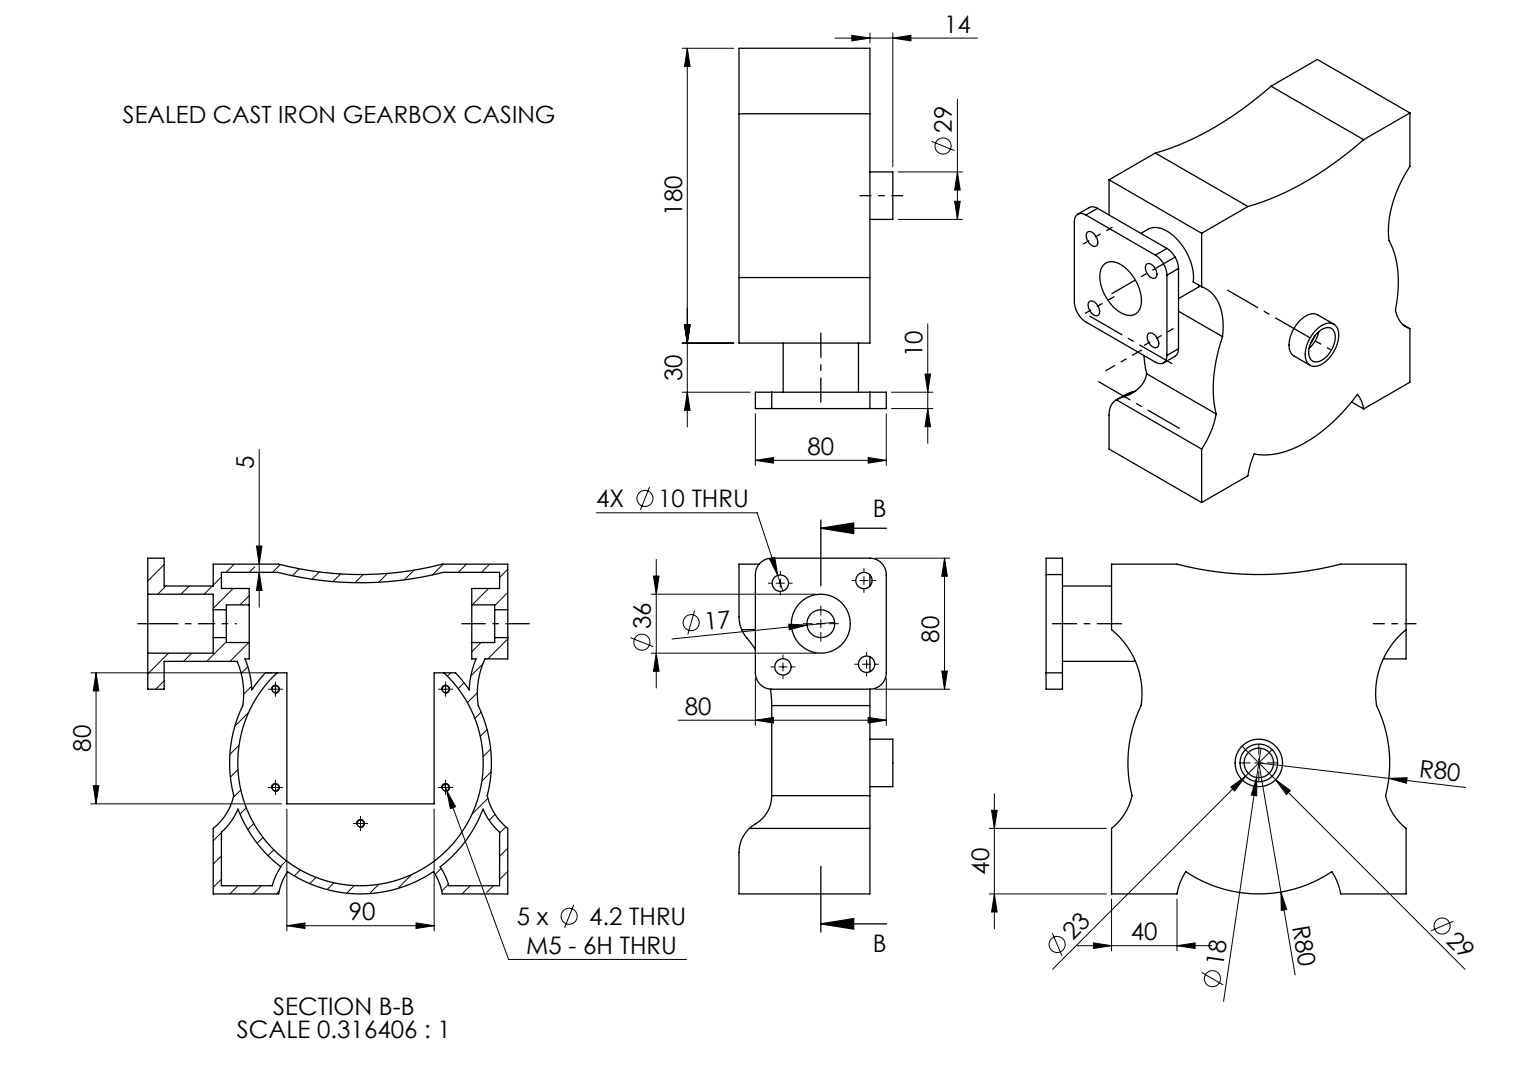
ISO-10303-21;
HEADER;
FILE_DESCRIPTION (('STEP AP214'),
    '1' );
FILE_NAME ('Sealed Cast Iron Gearbox Casing.step',
    '2026-10-03T12:29:21',
    ( '' ),
    ( '' ),
    'SwSTEP 2.0',
    'SolidWorks 2026',
    '' );
FILE_SCHEMA (( 'AUTOMOTIVE_DESIGN' ));
ENDSEC;

DATA;
#3=ADVANCED_FACE ( 'NONE', ( #6649 ), #1884, .F. ) ;
#5=ADVANCED_FACE ( 'NONE', ( #12919 ), #11518, .F. ) ;
#6=DIRECTION ( 'NONE',  ( 0.000000000000000000, 0.000000000000000000, -1.000000000000000000 ) ) ;
#7=CARTESIAN_POINT ( 'NONE',  ( -30.00000000000000000, -42.57363661491096707, -71.38288848018790134 ) ) ;
#14=DIRECTION ( 'NONE',  ( -1.000000000000000000, 0.000000000000000000, 0.000000000000000000 ) ) ;
#17=CARTESIAN_POINT ( 'NONE',  ( 24.99999999999999645, -39.99999999999999289, 52.00000000000000000 ) ) ;
#20=CARTESIAN_POINT ( 'NONE',  ( 33.05469362121638000, -30.48475803102838100, 72.85691518208254536 ) ) ;
#22=( GEOMETRIC_REPRESENTATION_CONTEXT ( 3 ) GLOBAL_UNCERTAINTY_ASSIGNED_CONTEXT ( ( #13875 ) ) GLOBAL_UNIT_ASSIGNED_CONTEXT ( ( #2142, #14970, #8601 ) ) REPRESENTATION_CONTEXT ( 'NONE', 'WORKASPACE' ) );
#26=EDGE_CURVE ( 'NONE', #19472, #5238, #10237, .T. ) ;
#28=CARTESIAN_POINT ( 'NONE',  ( -30.00000000000000000, -85.00000000000000000, -1.040949779275250179E-14 ) ) ;
#32=VECTOR ( 'NONE', #14335, 1000.000000000000000 ) ;
#35=AXIS2_PLACEMENT_3D ( 'NONE', #14775, #17865, #16462 ) ;
#46=ORIENTED_EDGE ( 'NONE', *, *, #5820, .T. ) ;
#47=VECTOR ( 'NONE', #20298, 1000.000000000000000 ) ;
#48=DIRECTION ( 'NONE',  ( 0.000000000000000000, 0.000000000000000000, -1.000000000000000000 ) ) ;
#50=DIRECTION ( 'NONE',  ( 0.000000000000000000, 0.000000000000000000, -1.000000000000000000 ) ) ;
#51=CIRCLE ( 'NONE', #6813, 3.199999999999994404 ) ;
#55=ADVANCED_FACE ( 'NONE', ( #11330 ), #295, .T. ) ;
#59=CARTESIAN_POINT ( 'NONE',  ( 40.00000000000000711, 29.99999999999999289, -120.0000000000000142 ) ) ;
#84=DIRECTION ( 'NONE',  ( -1.000000000000000000, -0.000000000000000000, -0.000000000000000000 ) ) ;
#86=ADVANCED_FACE ( 'NONE', ( #9826 ), #1783, .F. ) ;
#90=DIRECTION ( 'NONE',  ( -0.000000000000000000, -0.000000000000000000, 1.000000000000000000 ) ) ;
#95=FACE_OUTER_BOUND ( 'NONE', #12969, .T. ) ;
#101=CARTESIAN_POINT ( 'NONE',  ( 24.99999999999999645, -39.99999999999999289, -52.00000000000000000 ) ) ;
#104=LINE ( 'NONE', #16119, #19750 ) ;
#106=AXIS2_PLACEMENT_3D ( 'NONE', #7113, #10104, #5421 ) ;
#112=CARTESIAN_POINT ( 'NONE',  ( -44.00000000000000000, -85.00000000000000000, -1.040949779275250179E-14 ) ) ;
#113=EDGE_LOOP ( 'NONE', ( #18072, #15084 ) ) ;
#120=DIRECTION ( 'NONE',  ( -0.000000000000000000, -0.000000000000000000, 1.000000000000000000 ) ) ;
#123=CARTESIAN_POINT ( 'NONE',  ( 44.16803006078449556, -9.910160788546479083, 83.48928124825249597 ) ) ;
#128=DIRECTION ( 'NONE',  ( 1.000000000000000000, 0.000000000000000000, 0.000000000000000000 ) ) ;
#129=AXIS2_PLACEMENT_3D ( 'NONE', #17795, #12823, #16096 ) ;
#130=DIRECTION ( 'NONE',  ( 0.000000000000000000, 0.000000000000000000, -1.000000000000000000 ) ) ;
#136=DIRECTION ( 'NONE',  ( 0.000000000000000000, 0.000000000000000000, -1.000000000000000000 ) ) ;
#149=VECTOR ( 'NONE', #9986, 1000.000000000000000 ) ;
#152=EDGE_CURVE ( 'NONE', #4283, #2747, #12613, .T. ) ;
#161=CARTESIAN_POINT ( 'NONE',  ( -21.25952603694473808, -3.390848217253789265, -82.75718265314235111 ) ) ;
#163=DIRECTION ( 'NONE',  ( 0.000000000000000000, 0.000000000000000000, -1.000000000000000000 ) ) ;
#166=EDGE_CURVE ( 'NONE', #18682, #10203, #2445, .T. ) ;
#172=DIRECTION ( 'NONE',  ( 0.000000000000000000, 0.000000000000000000, -1.000000000000000000 ) ) ;
#176=ORIENTED_EDGE ( 'NONE', *, *, #6087, .T. ) ;
#183=ORIENTED_EDGE ( 'NONE', *, *, #18142, .F. ) ;
#185=DIRECTION ( 'NONE',  ( 1.000000000000000000, 0.000000000000000000, 0.000000000000000000 ) ) ;
#192=DIRECTION ( 'NONE',  ( -1.000000000000000000, 0.000000000000000000, 0.000000000000000000 ) ) ;
#195=ORIENTED_EDGE ( 'NONE', *, *, #17248, .F. ) ;
#199=DIRECTION ( 'NONE',  ( 0.000000000000000000, 0.000000000000000000, 1.000000000000000000 ) ) ;
#205=DIRECTION ( 'NONE',  ( 0.000000000000000000, 0.000000000000000000, -1.000000000000000000 ) ) ;
#209=VECTOR ( 'NONE', #12697, 1000.000000000000114 ) ;
#210=EDGE_CURVE ( 'NONE', #9883, #2104, #5368, .T. ) ;
#211=DIRECTION ( 'NONE',  ( 1.000000000000000000, 0.000000000000000000, 0.000000000000000000 ) ) ;
#222=CARTESIAN_POINT ( 'NONE',  ( 30.00000000000000000, -99.99999999999998579, -52.00000000000000000 ) ) ;
#228=CARTESIAN_POINT ( 'NONE',  ( 50.00000000000000000, -110.0000000000000000, -45.00000000000000711 ) ) ;
#229=CARTESIAN_POINT ( 'NONE',  ( 31.94499812652455617, -34.25508116175669215, 72.04208363913775770 ) ) ;
#231=VERTEX_POINT ( 'NONE', #15440 ) ;
#236=ADVANCED_FACE ( 'NONE', ( #17031 ), #2519, .F. ) ;
#239=ORIENTED_EDGE ( 'NONE', *, *, #11369, .T. ) ;
#243=CARTESIAN_POINT ( 'NONE',  ( 31.48472450438898207, -112.5746437239468776, -80.05721278606669955 ) ) ;
#246=DIRECTION ( 'NONE',  ( -1.000000000000000000, 0.000000000000000000, 0.000000000000000000 ) ) ;
#259=EDGE_LOOP ( 'NONE', ( #20380, #378, #6522, #9090 ) ) ;
#262=CARTESIAN_POINT ( 'NONE',  ( 0.000000000000000000, 0.000000000000000000, 84.99999999999998579 ) ) ;
#269=DIRECTION ( 'NONE',  ( -1.000000000000000000, 0.000000000000000000, 0.000000000000000000 ) ) ;
#274=EDGE_CURVE ( 'NONE', #4186, #16423, #8543, .T. ) ;
#295=CYLINDRICAL_SURFACE ( 'NONE', #11260, 80.00000000000000000 ) ;
#296=EDGE_CURVE ( 'NONE', #10832, #9434, #9184, .T. ) ;
#303=ORIENTED_EDGE ( 'NONE', *, *, #14253, .T. ) ;
#307=ORIENTED_EDGE ( 'NONE', *, *, #11823, .T. ) ;
#321=DIRECTION ( 'NONE',  ( -1.000000000000000000, 0.000000000000000000, 0.000000000000000000 ) ) ;
#331=ORIENTED_EDGE ( 'NONE', *, *, #12503, .F. ) ;
#332=ORIENTED_EDGE ( 'NONE', *, *, #5820, .F. ) ;
#336=DIRECTION ( 'NONE',  ( 1.000000000000000000, 0.000000000000000000, 0.000000000000000000 ) ) ;
#342=CARTESIAN_POINT ( 'NONE',  ( 30.00000000000000000, -39.99999999999999289, -52.00000000000000000 ) ) ;
#343=ORIENTED_EDGE ( 'NONE', *, *, #19126, .T. ) ;
#359=DIRECTION ( 'NONE',  ( -0.000000000000000000, -1.000000000000000000, -0.000000000000000000 ) ) ;
#360=VECTOR ( 'NONE', #15398, 1000.000000000000000 ) ;
#363=DIRECTION ( 'NONE',  ( -1.000000000000000000, 0.000000000000000000, 0.000000000000000000 ) ) ;
#375=ORIENTED_EDGE ( 'NONE', *, *, #7332, .F. ) ;
#376=DIRECTION ( 'NONE',  ( 0.000000000000000000, 0.000000000000000000, -1.000000000000000000 ) ) ;
#378=ORIENTED_EDGE ( 'NONE', *, *, #18023, .T. ) ;
#385=AXIS2_PLACEMENT_3D ( 'NONE', #5569, #16920, #8861 ) ;
#391=FACE_BOUND ( 'NONE', #20016, .T. ) ;
#398=CIRCLE ( 'NONE', #17331, 10.00000000000000178 ) ;
#405=VERTEX_POINT ( 'NONE', #11404 ) ;
#408=CARTESIAN_POINT ( 'NONE',  ( 48.80907113954126686, -2.531514235868165041, -83.66807691527674251 ) ) ;
#410=EDGE_CURVE ( 'NONE', #20805, #2701, #9805, .T. ) ;
#411=CARTESIAN_POINT ( 'NONE',  ( -27.96694501150314593, -24.74873734152930993, -120.0000000000000142 ) ) ;
#414=B_SPLINE_CURVE_WITH_KNOTS ( 'NONE', 3,
 ( #19492, #9752, #16310, #4765, #6760, #9842, #11534, #9653 ),
 .UNSPECIFIED., .F., .F.,
 ( 4, 2, 2, 4 ),
 ( 0.000000000000000000, 0.005433550342329228865, 0.008150325513493860211, 0.01086710068465849069 ),
 .UNSPECIFIED. ) ;
#426=EDGE_LOOP ( 'NONE', ( #46, #12533, #18701, #17009 ) ) ;
#429=PLANE ( 'NONE',  #8031 ) ;
#433=EDGE_CURVE ( 'NONE', #17850, #17173, #15609, .T. ) ;
#436=ADVANCED_FACE ( 'NONE', ( #3137 ), #6413, .T. ) ;
#438=CARTESIAN_POINT ( 'NONE',  ( 33.67895669406915715, -28.64151946020273343, 73.35365590739139918 ) ) ;
#442=CIRCLE ( 'NONE', #19390, 2.099999999999997868 ) ;
#446=AXIS2_PLACEMENT_3D ( 'NONE', #8844, #4070, #16804 ) ;
#447=PRESENTATION_STYLE_ASSIGNMENT (( #16544 ) ) ;
#449=DIRECTION ( 'NONE',  ( 0.000000000000000000, 0.000000000000000000, -1.000000000000000000 ) ) ;
#455=DIRECTION ( 'NONE',  ( 1.000000000000000000, 0.000000000000000000, 0.000000000000000000 ) ) ;
#458=ORIENTED_EDGE ( 'NONE', *, *, #13711, .F. ) ;
#472=DIRECTION ( 'NONE',  ( -1.000000000000000000, 0.000000000000000000, 0.000000000000000000 ) ) ;
#474=AXIS2_PLACEMENT_3D ( 'NONE', #7316, #10187, #8701 ) ;
#476=AXIS2_PLACEMENT_3D ( 'NONE', #11866, #6887, #5498 ) ;
#492=AXIS2_PLACEMENT_3D ( 'NONE', #3114, #20504, #7782 ) ;
#495=CARTESIAN_POINT ( 'NONE',  ( 50.00000000000000000, 36.35083268962915781, -50.00000000000000000 ) ) ;
#508=DIRECTION ( 'NONE',  ( 0.000000000000000000, 0.000000000000000000, -1.000000000000000000 ) ) ;
#512=DIRECTION ( 'NONE',  ( -0.000000000000000000, 0.000000000000000000, 1.000000000000000000 ) ) ;
#515=ORIENTED_EDGE ( 'NONE', *, *, #13376, .F. ) ;
#519=ORIENTED_EDGE ( 'NONE', *, *, #3660, .T. ) ;
#524=CYLINDRICAL_SURFACE ( 'NONE', #10905, 80.00000000000000000 ) ;
#534=ADVANCED_FACE ( 'NONE', ( #19430 ), #11383, .F. ) ;
#539=CARTESIAN_POINT ( 'NONE',  ( 0.000000000000000000, 0.000000000000000000, -120.0000000000000142 ) ) ;
#544=DIRECTION ( 'NONE',  ( 0.000000000000000000, 0.000000000000000000, -1.000000000000000000 ) ) ;
#548=EDGE_CURVE ( 'NONE', #12159, #1568, #1422, .T. ) ;
#549=ORIENTED_EDGE ( 'NONE', *, *, #7060, .T. ) ;
#552=DIRECTION ( 'NONE',  ( 0.000000000000000000, -0.000000000000000000, 1.000000000000000000 ) ) ;
#554=EDGE_CURVE ( 'NONE', #1571, #4727, #3426, .T. ) ;
#557=LINE ( 'NONE', #11880, #11849 ) ;
#560=CARTESIAN_POINT ( 'NONE',  ( -44.00000000000000000, -85.00000000000000000, -14.50000000000000533 ) ) ;
#564=FACE_OUTER_BOUND ( 'NONE', #13636, .T. ) ;
#569=ORIENTED_EDGE ( 'NONE', *, *, #18170, .F. ) ;
#572=EDGE_CURVE ( 'NONE', #17279, #5928, #1748, .T. ) ;
#573=CARTESIAN_POINT ( 'NONE',  ( 44.19470160754491417, -125.5384278435233085, 83.11447728151287606 ) ) ;
#574=CARTESIAN_POINT ( 'NONE',  ( 30.00000000000000000, 4.299168419249259188, -90.00000000000001421 ) ) ;
#577=VECTOR ( 'NONE', #11848, 1000.000000000000000 ) ;
#578=CARTESIAN_POINT ( 'NONE',  ( 50.00000000000000000, -30.00000000000000711, 44.99999999999998579 ) ) ;
#582=CARTESIAN_POINT ( 'NONE',  ( 0.000000000000000000, 0.000000000000000000, -81.99999999999998579 ) ) ;
#584=ORIENTED_EDGE ( 'NONE', *, *, #5461, .T. ) ;
#585=EDGE_CURVE ( 'NONE', #14577, #18338, #19669, .T. ) ;
#586=CARTESIAN_POINT ( 'NONE',  ( 30.00000000000000000, -85.00000000000000000, 79.99999999999998579 ) ) ;
#589=CARTESIAN_POINT ( 'NONE',  ( -10.25561400234657583, -18.90011081285701877, -71.73813932909898483 ) ) ;
#590=ORIENTED_EDGE ( 'NONE', *, *, #11130, .F. ) ;
#591=AXIS2_PLACEMENT_3D ( 'NONE', #11419, #8126, #19460 ) ;
#594=CARTESIAN_POINT ( 'NONE',  ( 0.000000000000000000, 0.000000000000000000, 81.99999999999998579 ) ) ;
#604=DIRECTION ( 'NONE',  ( 0.000000000000000000, 1.059758341687649568E-14, -1.000000000000000000 ) ) ;
#621=ORIENTED_EDGE ( 'NONE', *, *, #10925, .T. ) ;
#622=DIRECTION ( 'NONE',  ( 1.000000000000000000, 0.000000000000000000, 0.000000000000000000 ) ) ;
#631=EDGE_CURVE ( 'NONE', #10778, #3180, #16303, .T. ) ;
#639=ORIENTED_EDGE ( 'NONE', *, *, #9100, .F. ) ;
#641=ORIENTED_EDGE ( 'NONE', *, *, #12600, .T. ) ;
#642=PLANE ( 'NONE',  #16291 ) ;
#652=DIRECTION ( 'NONE',  ( -1.000000000000000000, 0.000000000000000000, 0.000000000000000000 ) ) ;
#658=LINE ( 'NONE', #7216, #18688 ) ;
#661=CARTESIAN_POINT ( 'NONE',  ( 10.15192380093072089, -18.95599582743659539, 71.71153801002559192 ) ) ;
#668=EDGE_CURVE ( 'NONE', #4597, #15761, #8490, .T. ) ;
#672=EDGE_CURVE ( 'NONE', #12901, #12906, #658, .T. ) ;
#682=CARTESIAN_POINT ( 'NONE',  ( 20.42938063014383943, -6.725612673823790466, -79.66382435179507127 ) ) ;
#685=DIRECTION ( 'NONE',  ( 0.000000000000000000, 0.000000000000000000, 1.000000000000000000 ) ) ;
#686=DIRECTION ( 'NONE',  ( -1.000000000000000000, 0.000000000000000000, 0.000000000000000000 ) ) ;
#687=ORIENTED_EDGE ( 'NONE', *, *, #3710, .F. ) ;
#690=LINE ( 'NONE', #15423, #17999 ) ;
#695=ORIENTED_EDGE ( 'NONE', *, *, #18063, .F. ) ;
#699=FACE_OUTER_BOUND ( 'NONE', #426, .T. ) ;
#717=ORIENTED_EDGE ( 'NONE', *, *, #10249, .T. ) ;
#718=ORIENTED_EDGE ( 'NONE', *, *, #18889, .F. ) ;
#719=CARTESIAN_POINT ( 'NONE',  ( 24.74873734152916072, 24.74873734152916072, -120.0000000000000142 ) ) ;
#732=ADVANCED_FACE ( 'NONE', ( #564 ), #19740, .T. ) ;
#734=CARTESIAN_POINT ( 'NONE',  ( 10.00000000000000178, -160.0000000000000000, 66.80000000000001137 ) ) ;
#738=DIRECTION ( 'NONE',  ( 1.000000000000000000, 0.000000000000000000, 0.000000000000000000 ) ) ;
#744=ORIENTED_EDGE ( 'NONE', *, *, #12088, .F. ) ;
#751=CYLINDRICAL_SURFACE ( 'NONE', #17029, 3.199999999999994404 ) ;
#753=VECTOR ( 'NONE', #11122, 1000.000000000000000 ) ;
#767=AXIS2_PLACEMENT_3D ( 'NONE', #7150, #12247, #15530 ) ;
#792=CARTESIAN_POINT ( 'NONE',  ( -6.110423144575273469, -20.66992657861278460, -70.93137971084412641 ) ) ;
#793=ORIENTED_EDGE ( 'NONE', *, *, #6745, .F. ) ;
#801=ORIENTED_EDGE ( 'NONE', *, *, #7784, .T. ) ;
#803=EDGE_CURVE ( 'NONE', #3394, #12901, #13494, .T. ) ;
#807=AXIS2_PLACEMENT_3D ( 'NONE', #10287, #13262, #8585 ) ;
#809=CARTESIAN_POINT ( 'NONE',  ( -30.00000000000000000, -97.49621075554985339, 111.6458212409894486 ) ) ;
#810=CARTESIAN_POINT ( 'NONE',  ( -30.00000000000000000, -85.00000000000000000, -1.040949779275250179E-14 ) ) ;
#818=ADVANCED_FACE ( 'NONE', ( #18673 ), #15389, .F. ) ;
#820=EDGE_CURVE ( 'NONE', #7631, #6575, #13600, .T. ) ;
#823=ORIENTED_EDGE ( 'NONE', *, *, #14598, .T. ) ;
#824=EDGE_CURVE ( 'NONE', #19846, #5684, #5131, .T. ) ;
#829=CARTESIAN_POINT ( 'NONE',  ( 1.577030005767653176, -22.95872380089934950, -75.39090623211717457 ) ) ;
#830=ORIENTED_EDGE ( 'NONE', *, *, #2623, .F. ) ;
#831=DIRECTION ( 'NONE',  ( -0.000000000000000000, -0.000000000000000000, 1.000000000000000000 ) ) ;
#834=VERTEX_POINT ( 'NONE', #15705 ) ;
#837=FACE_BOUND ( 'NONE', #113, .T. ) ;
#839=LINE ( 'NONE', #10479, #15988 ) ;
#844=CARTESIAN_POINT ( 'NONE',  ( 30.00000000000000000, -99.99999999999998579, -49.90000000000000568 ) ) ;
#855=DIRECTION ( 'NONE',  ( 0.000000000000000000, -1.000000000000000000, 0.000000000000000000 ) ) ;
#858=ORIENTED_EDGE ( 'NONE', *, *, #9285, .F. ) ;
#860=DIRECTION ( 'NONE',  ( -1.000000000000000000, 0.000000000000000000, 0.000000000000000000 ) ) ;
#872=DIRECTION ( 'NONE',  ( 0.000000000000000000, 0.000000000000000000, -1.000000000000000000 ) ) ;
#873=CIRCLE ( 'NONE', #3566, 39.99999999999999289 ) ;
#876=CARTESIAN_POINT ( 'NONE',  ( 12.05832282520465704, -17.81513111787451464, 72.26823280878556943 ) ) ;
#878=EDGE_LOOP ( 'NONE', ( #15752, #1382 ) ) ;
#883=FACE_BOUND ( 'NONE', #8855, .T. ) ;
#884=DIRECTION ( 'NONE',  ( -0.000000000000000000, -0.000000000000000000, 1.000000000000000000 ) ) ;
#886=DIRECTION ( 'NONE',  ( 1.000000000000000000, 0.000000000000000000, 0.000000000000000000 ) ) ;
#888=CARTESIAN_POINT ( 'NONE',  ( 30.00000000000000355, -139.6410161513775563, 85.00000000000000000 ) ) ;
#895=ADVANCED_FACE ( 'NONE', ( #10513 ), #7536, .T. ) ;
#900=CARTESIAN_POINT ( 'NONE',  ( 10.00000000000000178, -164.9999999999999716, -70.00000000000000000 ) ) ;
#902=CARTESIAN_POINT ( 'NONE',  ( -13.32881486730456366, -16.88549087568889462, -72.74798471664084332 ) ) ;
#903=EDGE_LOOP ( 'NONE', ( #239, #12883, #15311, #19138, #7059, #15330, #9122, #10048, #7226 ) ) ;
#906=DIRECTION ( 'NONE',  ( -0.000000000000000000, -0.000000000000000000, 1.000000000000000000 ) ) ;
#909=LINE ( 'NONE', #7361, #12285 ) ;
#912=LINE ( 'NONE', #2704, #7153 ) ;
#914=ORIENTED_EDGE ( 'NONE', *, *, #6745, .T. ) ;
#916=CARTESIAN_POINT ( 'NONE',  ( 30.00000000000000000, -105.0000000000000000, 72.35596062816881613 ) ) ;
#922=ADVANCED_FACE ( 'NONE', ( #4365 ), #2675, .F. ) ;
#927=ORIENTED_EDGE ( 'NONE', *, *, #11369, .F. ) ;
#933=DIRECTION ( 'NONE',  ( 0.000000000000000000, 0.000000000000000000, -1.000000000000000000 ) ) ;
#944=B_SPLINE_CURVE_WITH_KNOTS ( 'NONE', 3,
 ( #16979, #3938, #20368, #5853, #573, #12328, #12116, #5424 ),
 .UNSPECIFIED., .F., .F.,
 ( 4, 2, 2, 4 ),
 ( 0.000000000000000000, 0.004496536736660343599, 0.006744805104990527975, 0.008993073473320711483 ),
 .UNSPECIFIED. ) ;
#945=AXIS2_PLACEMENT_3D ( 'NONE', #809, #7256, #13736 ) ;
#952=FACE_OUTER_BOUND ( 'NONE', #13338, .T. ) ;
#957=CARTESIAN_POINT ( 'NONE',  ( -21.18805271706017379, -3.649167310370820871, 90.00000000000000000 ) ) ;
#968=ORIENTED_EDGE ( 'NONE', *, *, #17940, .F. ) ;
#977=DIRECTION ( 'NONE',  ( -1.000000000000000000, 0.000000000000000000, 0.000000000000000000 ) ) ;
#982=CARTESIAN_POINT ( 'NONE',  ( 41.41808208302013128, -123.1392381480534226, -87.79662768828312380 ) ) ;
#991=ORIENTED_EDGE ( 'NONE', *, *, #19974, .T. ) ;
#993=ORIENTED_EDGE ( 'NONE', *, *, #14530, .T. ) ;
#996=CARTESIAN_POINT ( 'NONE',  ( -24.99999999999999289, -1.326995226329868993, -84.99999999999998579 ) ) ;
#1005=CARTESIAN_POINT ( 'NONE',  ( -24.99999999999999289, -148.4917293642369600, 48.67032260359988527 ) ) ;
#1020=AXIS2_PLACEMENT_3D ( 'NONE', #11935, #4312, #18410 ) ;
#1021=CARTESIAN_POINT ( 'NONE',  ( -23.00000000000000000, 2.816687638038912352E-15, -130.0000000000000000 ) ) ;
#1027=DIRECTION ( 'NONE',  ( -0.000000000000000000, 0.000000000000000000, -1.000000000000000000 ) ) ;
#1038=ADVANCED_FACE ( 'NONE', ( #7857 ), #11357, .F. ) ;
#1049=DIRECTION ( 'NONE',  ( 1.000000000000000000, 0.000000000000000000, 0.000000000000000000 ) ) ;
#1060=DIRECTION ( 'NONE',  ( 0.000000000000000000, 0.000000000000000000, -1.000000000000000000 ) ) ;
#1062=DIRECTION ( 'NONE',  ( 0.000000000000000000, 0.000000000000000000, -1.000000000000000000 ) ) ;
#1074=VECTOR ( 'NONE', #9967, 1000.000000000000000 ) ;
#1078=AXIS2_PLACEMENT_3D ( 'NONE', #20638, #18751, #15770 ) ;
#1087=EDGE_CURVE ( 'NONE', #13160, #12463, #19294, .T. ) ;
#1091=ORIENTED_EDGE ( 'NONE', *, *, #10308, .F. ) ;
#1096=CIRCLE ( 'NONE', #1020, 8.500000000000000000 ) ;
#1102=DIRECTION ( 'NONE',  ( -1.000000000000000000, 0.000000000000000000, 0.000000000000000000 ) ) ;
#1105=CARTESIAN_POINT ( 'NONE',  ( -24.99999999999999289, -85.00000000000000000, -1.040949779275250179E-14 ) ) ;
#1107=VECTOR ( 'NONE', #1062, 1000.000000000000000 ) ;
#1108=AXIS2_PLACEMENT_3D ( 'NONE', #14210, #12619, #4013 ) ;
#1112=FACE_OUTER_BOUND ( 'NONE', #19436, .T. ) ;
#1115=FACE_OUTER_BOUND ( 'NONE', #5139, .T. ) ;
#1127=VERTEX_POINT ( 'NONE', #13365 ) ;
#1133=DIRECTION ( 'NONE',  ( 0.000000000000000000, 0.000000000000000000, -1.000000000000000000 ) ) ;
#1135=LINE ( 'NONE', #15949, #12648 ) ;
#1139=ORIENTED_EDGE ( 'NONE', *, *, #7007, .F. ) ;
#1140=CIRCLE ( 'NONE', #15346, 21.50000000000000000 ) ;
#1149=CARTESIAN_POINT ( 'NONE',  ( 30.00000000000000000, -85.00000000000000000, -1.040949779275250179E-14 ) ) ;
#1155=VECTOR ( 'NONE', #3414, 1000.000000000000000 ) ;
#1158=AXIS2_PLACEMENT_3D ( 'NONE', #9951, #6764, #14839 ) ;
#1163=DIRECTION ( 'NONE',  ( -1.000000000000000000, -0.000000000000000000, -0.000000000000000000 ) ) ;
#1180=DIRECTION ( 'NONE',  ( 0.000000000000000000, 0.000000000000000000, -1.000000000000000000 ) ) ;
#1185=VECTOR ( 'NONE', #19710, 1000.000000000000000 ) ;
#1186=CARTESIAN_POINT ( 'NONE',  ( 32.16538072331778864, -33.51036596020169611, -72.20447320033530048 ) ) ;
#1189=VERTEX_POINT ( 'NONE', #3697 ) ;
#1192=CYLINDRICAL_SURFACE ( 'NONE', #2080, 18.00000000000000000 ) ;
#1197=CARTESIAN_POINT ( 'NONE',  ( 0.000000000000000000, 0.000000000000000000, -90.00000000000000000 ) ) ;
#1198=DIRECTION ( 'NONE',  ( 0.000000000000000000, 0.000000000000000000, -1.000000000000000000 ) ) ;
#1209=ORIENTED_EDGE ( 'NONE', *, *, #12607, .T. ) ;
#1211=CARTESIAN_POINT ( 'NONE',  ( -25.00000000000000000, -30.00000000000000711, 58.09475019311124555 ) ) ;
#1213=VERTEX_POINT ( 'NONE', #19915 ) ;
#1214=DIRECTION ( 'NONE',  ( 1.000000000000000000, -0.000000000000000000, -0.000000000000000000 ) ) ;
#1219=EDGE_CURVE ( 'NONE', #4158, #16611, #3452, .T. ) ;
#1222=EDGE_CURVE ( 'NONE', #12434, #19457, #19607, .T. ) ;
#1224=VECTOR ( 'NONE', #20821, 1000.000000000000000 ) ;
#1228=CARTESIAN_POINT ( 'NONE',  ( 30.00000000000000000, -30.00000000000000711, -50.99019513592786268 ) ) ;
#1234=DIRECTION ( 'NONE',  ( 0.000000000000000000, 0.000000000000000000, -1.000000000000000000 ) ) ;
#1238=EDGE_LOOP ( 'NONE', ( #176, #20104, #6054, #11712 ) ) ;
#1242=CARTESIAN_POINT ( 'NONE',  ( 33.96219957007294710, -116.9571213503516987, 76.69693868221141031 ) ) ;
#1245=DIRECTION ( 'NONE',  ( 0.000000000000000000, 0.000000000000000000, -1.000000000000000000 ) ) ;
#1252=CARTESIAN_POINT ( 'NONE',  ( 10.80938043796751558, -18.58836422458828608, 77.51093294648217125 ) ) ;
#1259=VECTOR ( 'NONE', #13520, 1000.000000000000000 ) ;
#1265=CARTESIAN_POINT ( 'NONE',  ( -22.70866746290765903, -3.649167310370807105, -90.00000000000000000 ) ) ;
#1266=CARTESIAN_POINT ( 'NONE',  ( 40.00000000000000711, 29.99999999999999289, -120.0000000000000142 ) ) ;
#1273=CYLINDRICAL_SURFACE ( 'NONE', #6149, 21.50000000000000000 ) ;
#1274=CARTESIAN_POINT ( 'NONE',  ( 50.00000000000000000, 31.35083268962918979, -84.99999999999998579 ) ) ;
#1277=VECTOR ( 'NONE', #14393, 1000.000000000000000 ) ;
#1283=VECTOR ( 'NONE', #512, 1000.000000000000000 ) ;
#1286=CARTESIAN_POINT ( 'NONE',  ( 30.00000000000000000, -99.99999999999998579, -49.89999999999999858 ) ) ;
#1289=CARTESIAN_POINT ( 'NONE',  ( -44.00000000000000000, -85.00000000000000000, -1.040949779275250179E-14 ) ) ;
#1290=EDGE_LOOP ( 'NONE', ( #10169, #20048, #12447, #7217 ) ) ;
#1299=DIRECTION ( 'NONE',  ( -1.000000000000000000, 0.000000000000000000, 0.000000000000000000 ) ) ;
#1301=VECTOR ( 'NONE', #16668, 1000.000000000000000 ) ;
#1307=CARTESIAN_POINT ( 'NONE',  ( -30.00000000000000000, -105.0000000000000426, 77.45966692414833688 ) ) ;
#1310=DIRECTION ( 'NONE',  ( 0.000000000000000000, 0.000000000000000000, -1.000000000000000000 ) ) ;
#1313=CARTESIAN_POINT ( 'NONE',  ( 20.90734068544160706, -5.044436930659520257, 81.16927884214385358 ) ) ;
#1318=PLANE ( 'NONE',  #3965 ) ;
#1319=DIRECTION ( 'NONE',  ( -1.000000000000000000, -0.000000000000000000, -0.000000000000000000 ) ) ;
#1322=EDGE_CURVE ( 'NONE', #1127, #14263, #3129, .T. ) ;
#1333=CARTESIAN_POINT ( 'NONE',  ( 40.00000000000000711, -40.00000000000001421, -120.0000000000000142 ) ) ;
#1337=PLANE ( 'NONE',  #3265 ) ;
#1338=FACE_OUTER_BOUND ( 'NONE', #19789, .T. ) ;
#1348=EDGE_CURVE ( 'NONE', #4487, #10714, #7190, .T. ) ;
#1351=ORIENTED_EDGE ( 'NONE', *, *, #8849, .T. ) ;
#1353=CARTESIAN_POINT ( 'NONE',  ( 50.00000000000000000, 230.0000000000000000, -84.99999999999998579 ) ) ;
#1355=CARTESIAN_POINT ( 'NONE',  ( 4.941899431655324193, -20.93672964816920867, 76.30663123623098443 ) ) ;
#1359=EDGE_CURVE ( 'NONE', #1568, #8829, #15366, .T. ) ;
#1361=ORIENTED_EDGE ( 'NONE', *, *, #18493, .F. ) ;
#1364=ORIENTED_EDGE ( 'NONE', *, *, #13741, .T. ) ;
#1366=DIRECTION ( 'NONE',  ( -0.000000000000000000, -0.000000000000000000, 1.000000000000000000 ) ) ;
#1370=LINE ( 'NONE', #13867, #10372 ) ;
#1372=CARTESIAN_POINT ( 'NONE',  ( 0.000000000000000000, 0.000000000000000000, -68.00000000000000000 ) ) ;
#1373=CARTESIAN_POINT ( 'NONE',  ( 42.61160110135224244, -124.0569253416645665, 88.80170281571383839 ) ) ;
#1380=DIRECTION ( 'NONE',  ( -0.000000000000000000, -0.000000000000000000, 1.000000000000000000 ) ) ;
#1382=ORIENTED_EDGE ( 'NONE', *, *, #1219, .F. ) ;
#1394=CARTESIAN_POINT ( 'NONE',  ( 33.20850901831757795, -115.8985490652624435, -76.12077281629255765 ) ) ;
#1402=DIRECTION ( 'NONE',  ( 0.000000000000000000, -1.000000000000000000, 0.000000000000000000 ) ) ;
#1404=CARTESIAN_POINT ( 'NONE',  ( 50.00000000000000000, 230.0000000000000000, 0.000000000000000000 ) ) ;
#1405=ORIENTED_EDGE ( 'NONE', *, *, #20300, .T. ) ;
#1406=DIRECTION ( 'NONE',  ( 1.000000000000000000, 0.000000000000000000, 0.000000000000000000 ) ) ;
#1409=CARTESIAN_POINT ( 'NONE',  ( 20.76542986210400699, -5.602711969362187183, 80.65560201174187682 ) ) ;
#1410=CIRCLE ( 'NONE', #3427, 80.00000000000000000 ) ;
#1422=CIRCLE ( 'NONE', #8837, 10.00000000000000178 ) ;
#1424=LINE ( 'NONE', #17631, #16707 ) ;
#1428=DIRECTION ( 'NONE',  ( -1.000000000000000000, 0.000000000000000000, 0.000000000000000000 ) ) ;
#1431=DIRECTION ( 'NONE',  ( 0.000000000000000000, 0.000000000000000000, -1.000000000000000000 ) ) ;
#1435=CARTESIAN_POINT ( 'NONE',  ( 50.00000000000000000, -159.9999999999999716, -85.00000000000000000 ) ) ;
#1443=CIRCLE ( 'NONE', #1108, 8.500000000000000000 ) ;
#1444=EDGE_CURVE ( 'NONE', #14263, #20655, #16203, .T. ) ;
#1445=ORIENTED_EDGE ( 'NONE', *, *, #14802, .T. ) ;
#1456=AXIS2_PLACEMENT_3D ( 'NONE', #495, #8223, #10027 ) ;
#1466=LINE ( 'NONE', #9410, #16845 ) ;
#1470=CARTESIAN_POINT ( 'NONE',  ( -19.56341920831713210, -12.11112665530244925, -81.72775504840210203 ) ) ;
#1472=CARTESIAN_POINT ( 'NONE',  ( 11.50000000000000000, 0.000000000000000000, 68.00000000000000000 ) ) ;
#1482=CIRCLE ( 'NONE', #13313, 20.00000000000000000 ) ;
#1491=LINE ( 'NONE', #4549, #19305 ) ;
#1495=DIRECTION ( 'NONE',  ( 1.734723475976806848E-16, 1.000000000000000000, 0.000000000000000000 ) ) ;
#1501=CARTESIAN_POINT ( 'NONE',  ( 50.00000000000000000, 31.35083268962916137, 50.63110039191614220 ) ) ;
#1505=DIRECTION ( 'NONE',  ( -1.000000000000000000, 0.000000000000000000, 0.000000000000000000 ) ) ;
#1522=CARTESIAN_POINT ( 'NONE',  ( 50.00000000000000000, 31.35083268962916137, -50.63110039191615641 ) ) ;
#1523=ORIENTED_EDGE ( 'NONE', *, *, #14301, .F. ) ;
#1532=FACE_OUTER_BOUND ( 'NONE', #6468, .T. ) ;
#1543=ORIENTED_EDGE ( 'NONE', *, *, #11308, .F. ) ;
#1545=FACE_OUTER_BOUND ( 'NONE', #6841, .T. ) ;
#1546=CYLINDRICAL_SURFACE ( 'NONE', #492, 11.50000000000000000 ) ;
#1547=EDGE_LOOP ( 'NONE', ( #5502, #13967, #18931, #4600 ) ) ;
#1550=AXIS2_PLACEMENT_3D ( 'NONE', #2111, #8569, #15046 ) ;
#1554=CARTESIAN_POINT ( 'NONE',  ( 36.52125820097372610, -119.8000680387651187, 78.43373391519315874 ) ) ;
#1556=DIRECTION ( 'NONE',  ( -1.000000000000000000, 0.000000000000000000, 0.000000000000000000 ) ) ;
#1560=DIRECTION ( 'NONE',  ( -8.673617379884035472E-17, 1.000000000000000000, 0.000000000000000000 ) ) ;
#1564=CARTESIAN_POINT ( 'NONE',  ( 15.98236128136674949, -14.38466504862504358, 80.08563004779874461 ) ) ;
#1568=VERTEX_POINT ( 'NONE', #17489 ) ;
#1571=VERTEX_POINT ( 'NONE', #2966 ) ;
#1572=FACE_OUTER_BOUND ( 'NONE', #15707, .T. ) ;
#1573=AXIS2_PLACEMENT_3D ( 'NONE', #14225, #20577, #1198 ) ;
#1577=CARTESIAN_POINT ( 'NONE',  ( 50.00000000000000000, -160.0000000000000000, 0.000000000000000000 ) ) ;
#1585=VECTOR ( 'NONE', #7418, 1000.000000000000000 ) ;
#1595=AXIS2_PLACEMENT_3D ( 'NONE', #3914, #8901, #10179 ) ;
#1599=ADVANCED_FACE ( 'NONE', ( #13730, #12239 ), #7248, .T. ) ;
#1601=AXIS2_PLACEMENT_3D ( 'NONE', #888, #7553, #4483 ) ;
#1604=CARTESIAN_POINT ( 'NONE',  ( 0.000000000000000000, 0.000000000000000000, 68.00000000000000000 ) ) ;
#1605=CIRCLE ( 'NONE', #20184, 40.00000000000000000 ) ;
#1606=ORIENTED_EDGE ( 'NONE', *, *, #4835, .F. ) ;
#1613=DIRECTION ( 'NONE',  ( 0.000000000000000000, 0.000000000000000000, -1.000000000000000000 ) ) ;
#1614=EDGE_CURVE ( 'NONE', #20241, #9722, #13622, .T. ) ;
#1619=DIRECTION ( 'NONE',  ( -1.000000000000000000, -0.000000000000000000, -0.000000000000000000 ) ) ;
#1623=VECTOR ( 'NONE', #9712, 1000.000000000000000 ) ;
#1631=VERTEX_POINT ( 'NONE', #1787 ) ;
#1638=DIRECTION ( 'NONE',  ( 1.000000000000000000, -0.000000000000000000, -0.000000000000000000 ) ) ;
#1639=CIRCLE ( 'NONE', #10071, 14.49999999999999467 ) ;
#1646=EDGE_CURVE ( 'NONE', #3206, #4597, #5057, .T. ) ;
#1648=LINE ( 'NONE', #13177, #18750 ) ;
#1649=LINE ( 'NONE', #1737, #19416 ) ;
#1656=VERTEX_POINT ( 'NONE', #2285 ) ;
#1658=ORIENTED_EDGE ( 'NONE', *, *, #7260, .T. ) ;
#1659=CARTESIAN_POINT ( 'NONE',  ( 35.31732902261087048, -118.6065303221148071, 77.66260182251970434 ) ) ;
#1660=DIRECTION ( 'NONE',  ( 0.000000000000000000, 0.000000000000000000, -1.000000000000000000 ) ) ;
#1663=ORIENTED_EDGE ( 'NONE', *, *, #3369, .F. ) ;
#1664=CARTESIAN_POINT ( 'NONE',  ( 50.00000000000000000, -164.9999999999999716, 50.00000000000001421 ) ) ;
#1675=CARTESIAN_POINT ( 'NONE',  ( -12.23225220234714072, -19.49129496293704733, -77.02726945203133369 ) ) ;
#1681=LINE ( 'NONE', #17450, #12263 ) ;
#1686=FACE_OUTER_BOUND ( 'NONE', #14854, .T. ) ;
#1688=DIRECTION ( 'NONE',  ( 0.000000000000000000, 0.000000000000000000, -1.000000000000000000 ) ) ;
#1694=CARTESIAN_POINT ( 'NONE',  ( 30.18435758154164006, -45.05736527963534144, 66.43021625834032307 ) ) ;
#1698=DIRECTION ( 'NONE',  ( -0.000000000000000000, -0.000000000000000000, 1.000000000000000000 ) ) ;
#1699=ORIENTED_EDGE ( 'NONE', *, *, #11165, .T. ) ;
#1703=CIRCLE ( 'NONE', #8439, 54.99999999999999289 ) ;
#1705=DIRECTION ( 'NONE',  ( 0.000000000000000000, 1.000000000000000000, 0.000000000000000000 ) ) ;
#1710=CARTESIAN_POINT ( 'NONE',  ( 0.000000000000000000, 0.000000000000000000, 68.00000000000000000 ) ) ;
#1711=EDGE_CURVE ( 'NONE', #1631, #18530, #909, .T. ) ;
#1712=EDGE_LOOP ( 'NONE', ( #16835, #8897, #8810, #11295 ) ) ;
#1716=DIRECTION ( 'NONE',  ( 1.000000000000000000, -0.000000000000000000, -0.000000000000000000 ) ) ;
#1718=DIRECTION ( 'NONE',  ( 1.000000000000000000, 0.000000000000000000, 0.000000000000000000 ) ) ;
#1719=EDGE_LOOP ( 'NONE', ( #16206, #15412 ) ) ;
#1721=CARTESIAN_POINT ( 'NONE',  ( 30.43430782549248903, -42.57363661491096707, -66.38288848018790134 ) ) ;
#1724=VECTOR ( 'NONE', #19074, 1000.000000000000000 ) ;
#1728=CIRCLE ( 'NONE', #11862, 23.00000000000000000 ) ;
#1737=CARTESIAN_POINT ( 'NONE',  ( 50.00000000000000000, -172.4842959289096598, 69.62001590667014739 ) ) ;
#1739=DIRECTION ( 'NONE',  ( -1.000000000000000000, 0.000000000000000000, 0.000000000000000000 ) ) ;
#1745=VERTEX_POINT ( 'NONE', #18821 ) ;
#1748=CIRCLE ( 'NONE', #16288, 8.500000000000000000 ) ;
#1752=VECTOR ( 'NONE', #19396, 1000.000000000000000 ) ;
#1764=FACE_OUTER_BOUND ( 'NONE', #9147, .T. ) ;
#1769=CARTESIAN_POINT ( 'NONE',  ( 50.00000000000000000, 230.0000000000000000, 0.000000000000000000 ) ) ;
#1773=CARTESIAN_POINT ( 'NONE',  ( 24.99999999999999645, -84.99999999999998579, -75.00000000000002842 ) ) ;
#1776=CARTESIAN_POINT ( 'NONE',  ( -24.99999999999999289, -97.49621075554985339, -111.6458212409894486 ) ) ;
#1781=DIRECTION ( 'NONE',  ( -1.000000000000000000, 0.000000000000000000, -0.000000000000000000 ) ) ;
#1783=CYLINDRICAL_SURFACE ( 'NONE', #7525, 5.000000000000000888 ) ;
#1787=CARTESIAN_POINT ( 'NONE',  ( 45.76122707727121508, -127.3290820621008947, 85.00000000000000000 ) ) ;
#1789=CARTESIAN_POINT ( 'NONE',  ( 33.60460458983040155, -28.85220587458695007, 68.11375585025291457 ) ) ;
#1790=AXIS2_PLACEMENT_3D ( 'NONE', #4738, #6524, #17677 ) ;
#1791=ORIENTED_EDGE ( 'NONE', *, *, #20113, .T. ) ;
#1794=CARTESIAN_POINT ( 'NONE',  ( 45.22159793441013420, -8.673994507468389514, -84.62946326583126222 ) ) ;
#1802=FACE_OUTER_BOUND ( 'NONE', #15616, .T. ) ;
#1804=DIRECTION ( 'NONE',  ( 0.000000000000000000, 0.000000000000000000, -1.000000000000000000 ) ) ;
#1817=CARTESIAN_POINT ( 'NONE',  ( 23.00000000000000000, 0.000000000000000000, -130.0000000000000000 ) ) ;
#1819=ORIENTED_EDGE ( 'NONE', *, *, #13003, .F. ) ;
#1824=CARTESIAN_POINT ( 'NONE',  ( 30.00000000000000711, -49.00129691733391724, 71.78747447449033814 ) ) ;
#1827=DIRECTION ( 'NONE',  ( -1.000000000000000000, 0.000000000000000000, 0.000000000000000000 ) ) ;
#1833=DIRECTION ( 'NONE',  ( 1.000000000000000000, -0.000000000000000000, -0.000000000000000000 ) ) ;
#1838=EDGE_CURVE ( 'NONE', #14211, #9376, #17446, .T. ) ;
#1839=CYLINDRICAL_SURFACE ( 'NONE', #11990, 2.099999999999997868 ) ;
#1840=CARTESIAN_POINT ( 'NONE',  ( -26.35784117651625280, 26.35784117651607872, -120.0000000000000142 ) ) ;
#1842=CARTESIAN_POINT ( 'NONE',  ( 50.00000000000000000, -105.0000000000000000, -90.00000000000001421 ) ) ;
#1843=EDGE_LOOP ( 'NONE', ( #9622, #15187, #15160, #5443, #19277 ) ) ;
#1847=DIRECTION ( 'NONE',  ( 0.000000000000000000, 1.000000000000000000, 0.000000000000000000 ) ) ;
#1850=VERTEX_POINT ( 'NONE', #12560 ) ;
#1861=AXIS2_PLACEMENT_3D ( 'NONE', #10011, #19864, #6928 ) ;
#1865=DIRECTION ( 'NONE',  ( -0.000000000000000000, -1.000000000000000000, -0.000000000000000000 ) ) ;
#1874=ORIENTED_EDGE ( 'NONE', *, *, #17265, .T. ) ;
#1884=CYLINDRICAL_SURFACE ( 'NONE', #8531, 3.199999999999994404 ) ;
#1885=AXIS2_PLACEMENT_3D ( 'NONE', #10734, #17199, #2673 ) ;
#1889=CARTESIAN_POINT ( 'NONE',  ( 40.00000000000000711, 39.99999999999998579, -120.0000000000000142 ) ) ;
#1895=ORIENTED_EDGE ( 'NONE', *, *, #17550, .T. ) ;
#1916=CARTESIAN_POINT ( 'NONE',  ( 30.00000000000000000, -85.00000000000000000, -1.040949779275250179E-14 ) ) ;
#1917=ORIENTED_EDGE ( 'NONE', *, *, #14933, .F. ) ;
#1924=ORIENTED_EDGE ( 'NONE', *, *, #1087, .F. ) ;
#1926=CIRCLE ( 'NONE', #5641, 10.00000000000000178 ) ;
#1927=( LENGTH_UNIT ( ) NAMED_UNIT ( * ) SI_UNIT ( .MILLI., .METRE. ) );
#1932=AXIS2_PLACEMENT_3D ( 'NONE', #8446, #11944, #15028 ) ;
#1940=CARTESIAN_POINT ( 'NONE',  ( 50.00000000000000000, -110.0000000000000142, 44.99999999999999289 ) ) ;
#1946=EDGE_CURVE ( 'NONE', #12559, #405, #19541, .T. ) ;
#1947=CYLINDRICAL_SURFACE ( 'NONE', #13320, 8.999999999999994671 ) ;
#1951=CIRCLE ( 'NONE', #13119, 20.00000000000000000 ) ;
#1961=ORIENTED_EDGE ( 'NONE', *, *, #12432, .T. ) ;
#1962=DIRECTION ( 'NONE',  ( 0.000000000000000000, 0.000000000000000000, -1.000000000000000000 ) ) ;
#1964=DIRECTION ( 'NONE',  ( 1.000000000000000000, -0.000000000000000000, -0.000000000000000000 ) ) ;
#1969=DIRECTION ( 'NONE',  ( -0.000000000000000000, -0.000000000000000000, 1.000000000000000000 ) ) ;
#1972=EDGE_CURVE ( 'NONE', #15306, #1213, #5023, .T. ) ;
#1976=ORIENTED_EDGE ( 'NONE', *, *, #19342, .F. ) ;
#1978=ADVANCED_FACE ( 'NONE', ( #13186 ), #1947, .F. ) ;
#1981=DIRECTION ( 'NONE',  ( -1.000000000000000000, 2.309263891220325289E-14, 0.000000000000000000 ) ) ;
#1985=ORIENTED_EDGE ( 'NONE', *, *, #9043, .F. ) ;
#1991=EDGE_CURVE ( 'NONE', #3526, #20820, #8403, .T. ) ;
#1995=ORIENTED_EDGE ( 'NONE', *, *, #572, .T. ) ;
#1996=EDGE_CURVE ( 'NONE', #3964, #14529, #6525, .T. ) ;
#1997=CARTESIAN_POINT ( 'NONE',  ( 37.19682189084361568, -120.3881242644580709, 85.16117312608449197 ) ) ;
#1999=VERTEX_POINT ( 'NONE', #17648 ) ;
#2008=DIRECTION ( 'NONE',  ( 0.000000000000000000, -0.7812527682501556603, 0.6242147964454771714 ) ) ;
#2019=FACE_BOUND ( 'NONE', #2437, .T. ) ;
#2022=VECTOR ( 'NONE', #5978, 1000.000000000000000 ) ;
#2024=FACE_OUTER_BOUND ( 'NONE', #1238, .T. ) ;
#2033=CARTESIAN_POINT ( 'NONE',  ( 30.51289089809370125, -109.5903380226954056, -78.78839954496530140 ) ) ;
#2051=AXIS2_PLACEMENT_3D ( 'NONE', #20030, #8600, #15073 ) ;
#2053=CARTESIAN_POINT ( 'NONE',  ( 45.22159793441012710, -8.673994507468377080, 78.07221698934969822 ) ) ;
#2054=AXIS2_PLACEMENT_3D ( 'NONE', #16360, #6804, #14876 ) ;
#2056=EDGE_CURVE ( 'NONE', #405, #5157, #14981, .T. ) ;
#2066=ADVANCED_FACE ( 'NONE', ( #18160 ), #3724, .T. ) ;
#2069=FACE_OUTER_BOUND ( 'NONE', #7501, .T. ) ;
#2080=AXIS2_PLACEMENT_3D ( 'NONE', #5832, #17194, #12523 ) ;
#2081=EDGE_CURVE ( 'NONE', #11554, #20725, #11691, .T. ) ;
#2083=ORIENTED_EDGE ( 'NONE', *, *, #7957, .T. ) ;
#2086=AXIS2_PLACEMENT_3D ( 'NONE', #13971, #4530, #7604 ) ;
#2092=CARTESIAN_POINT ( 'NONE',  ( 30.00000000000000000, -105.0000000000000426, 77.45966692414833688 ) ) ;
#2097=VECTOR ( 'NONE', #11885, 1000.000000000000114 ) ;
#2101=ORIENTED_EDGE ( 'NONE', *, *, #16469, .T. ) ;
#2104=VERTEX_POINT ( 'NONE', #4042 ) ;
#2108=DIRECTION ( 'NONE',  ( 0.7071067811865436870, 0.4413865154835798221, 0.5524291302504504841 ) ) ;
#2110=EDGE_CURVE ( 'NONE', #7909, #19902, #2462, .T. ) ;
#2111=CARTESIAN_POINT ( 'NONE',  ( -24.99999999999999289, 230.0000000000000000, 0.000000000000000000 ) ) ;
#2121=CARTESIAN_POINT ( 'NONE',  ( 23.13963350654227824, -26.35784117651622793, -130.0000000000000000 ) ) ;
#2123=FACE_BOUND ( 'NONE', #12789, .T. ) ;
#2130=VERTEX_POINT ( 'NONE', #19941 ) ;
#2131=ORIENTED_EDGE ( 'NONE', *, *, #7332, .T. ) ;
#2133=AXIS2_PLACEMENT_3D ( 'NONE', #1776, #11421, #6635 ) ;
#2141=CYLINDRICAL_SURFACE ( 'NONE', #2051, 2.099999999999997868 ) ;
#2142=( LENGTH_UNIT ( ) NAMED_UNIT ( * ) SI_UNIT ( .MILLI., .METRE. ) );
#2144=CYLINDRICAL_SURFACE ( 'NONE', #16598, 20.00000000000000355 ) ;
#2146=ORIENTED_EDGE ( 'NONE', *, *, #554, .F. ) ;
#2149=VERTEX_POINT ( 'NONE', #10423 ) ;
#2151=CARTESIAN_POINT ( 'NONE',  ( -10.58466049171560464, -18.71773173394922196, 71.82544846116155668 ) ) ;
#2152=ORIENTED_EDGE ( 'NONE', *, *, #8330, .T. ) ;
#2160=VECTOR ( 'NONE', #14156, 1000.000000000000000 ) ;
#2163=CIRCLE ( 'NONE', #474, 21.50000000000000000 ) ;
#2164=CARTESIAN_POINT ( 'NONE',  ( 30.14578621226506172, -45.03195997035788167, -66.38288848018790134 ) ) ;
#2173=CARTESIAN_POINT ( 'NONE',  ( -13.88581415360054550, -16.42997871820715616, -72.99065141121242561 ) ) ;
#2196=CARTESIAN_POINT ( 'NONE',  ( 30.50907704923281472, -109.5730600679726052, 78.78220139038879211 ) ) ;
#2203=CARTESIAN_POINT ( 'NONE',  ( 50.00000000000000000, 230.0000000000000000, -85.00000000000000000 ) ) ;
#2211=EDGE_CURVE ( 'NONE', #1850, #5277, #5524, .T. ) ;
#2230=DIRECTION ( 'NONE',  ( 1.000000000000000000, -0.000000000000000000, -0.000000000000000000 ) ) ;
#2240=AXIS2_PLACEMENT_3D ( 'NONE', #11200, #16463, #4634 ) ;
#2241=DIRECTION ( 'NONE',  ( 0.000000000000000000, 0.000000000000000000, -1.000000000000000000 ) ) ;
#2244=CARTESIAN_POINT ( 'NONE',  ( 30.06750564394959824, -106.8813891955586257, -77.91416960582807860 ) ) ;
#2246=DIRECTION ( 'NONE',  ( 0.000000000000000000, 0.000000000000000000, -1.000000000000000000 ) ) ;
#2247=FACE_OUTER_BOUND ( 'NONE', #14955, .T. ) ;
#2258=CARTESIAN_POINT ( 'NONE',  ( 24.99999999999999289, -110.0000000000000142, 44.99999999999999289 ) ) ;
#2273=ORIENTED_EDGE ( 'NONE', *, *, #2295, .T. ) ;
#2275=CARTESIAN_POINT ( 'NONE',  ( 0.000000000000000000, 0.000000000000000000, -68.00000000000000000 ) ) ;
#2277=CARTESIAN_POINT ( 'NONE',  ( 4.119954785698654476, -21.10500016855060679, -70.74589478160186218 ) ) ;
#2278=ORIENTED_EDGE ( 'NONE', *, *, #15463, .T. ) ;
#2279=AXIS2_PLACEMENT_3D ( 'NONE', #4218, #17157, #20433 ) ;
#2282=CARTESIAN_POINT ( 'NONE',  ( 50.00000000000000000, -160.0000000000000000, 0.000000000000000000 ) ) ;
#2285=CARTESIAN_POINT ( 'NONE',  ( -32.96694501150314949, -24.74873734152930993, -120.0000000000000142 ) ) ;
#2289=ORIENTED_EDGE ( 'NONE', *, *, #19061, .F. ) ;
#2290=DIRECTION ( 'NONE',  ( -1.000000000000000000, -0.000000000000000000, -0.000000000000000000 ) ) ;
#2295=EDGE_CURVE ( 'NONE', #16235, #5869, #6885, .T. ) ;
#2296=CIRCLE ( 'NONE', #945, 34.99999999999999289 ) ;
#2297=DIRECTION ( 'NONE',  ( 1.000000000000000000, -0.000000000000000000, -0.000000000000000000 ) ) ;
#2300=ORIENTED_EDGE ( 'NONE', *, *, #631, .F. ) ;
#2306=VERTEX_POINT ( 'NONE', #14232 ) ;
#2309=EDGE_LOOP ( 'NONE', ( #16752, #9506 ) ) ;
#2311=ORIENTED_EDGE ( 'NONE', *, *, #10468, .F. ) ;
#2333=LINE ( 'NONE', #18133, #7581 ) ;
#2335=CARTESIAN_POINT ( 'NONE',  ( -31.35784117651625635, 26.35784117651607872, -120.0000000000000142 ) ) ;
#2338=ORIENTED_EDGE ( 'NONE', *, *, #11165, .F. ) ;
#2342=FACE_BOUND ( 'NONE', #2460, .T. ) ;
#2350=PLANE ( 'NONE',  #15362 ) ;
#2351=ORIENTED_EDGE ( 'NONE', *, *, #18142, .T. ) ;
#2357=ORIENTED_EDGE ( 'NONE', *, *, #4699, .T. ) ;
#2358=PRODUCT_DEFINITION ( 'UNKNOWN', '', #4244, #17267 ) ;
#2363=ORIENTED_EDGE ( 'NONE', *, *, #18967, .F. ) ;
#2365=EDGE_CURVE ( 'NONE', #9313, #2489, #17527, .T. ) ;
#2377=CARTESIAN_POINT ( 'NONE',  ( 3.744012722225332990, -21.17498532244396969, -70.71631193418077999 ) ) ;
#2382=ORIENTED_EDGE ( 'NONE', *, *, #17265, .F. ) ;
#2383=DIRECTION ( 'NONE',  ( 1.000000000000000000, 0.000000000000000000, 0.000000000000000000 ) ) ;
#2390=ORIENTED_EDGE ( 'NONE', *, *, #8242, .T. ) ;
#2401=CARTESIAN_POINT ( 'NONE',  ( -25.00000000000000000, -30.00000000000000711, 58.09475019311124555 ) ) ;
#2404=CARTESIAN_POINT ( 'NONE',  ( 31.31307953385777054, -112.1412981899224519, 79.85379371982303098 ) ) ;
#2408=VERTEX_POINT ( 'NONE', #17835 ) ;
#2422=VECTOR ( 'NONE', #9660, 1000.000000000000000 ) ;
#2425=DIRECTION ( 'NONE',  ( 0.000000000000000000, 0.000000000000000000, -1.000000000000000000 ) ) ;
#2426=ORIENTED_EDGE ( 'NONE', *, *, #18690, .F. ) ;
#2432=ORIENTED_EDGE ( 'NONE', *, *, #14802, .F. ) ;
#2434=ORIENTED_EDGE ( 'NONE', *, *, #13718, .F. ) ;
#2437=EDGE_LOOP ( 'NONE', ( #5886, #5732 ) ) ;
#2444=VECTOR ( 'NONE', #18332, 1000.000000000000000 ) ;
#2445=CIRCLE ( 'NONE', #14311, 39.99999999999999289 ) ;
#2449=FACE_OUTER_BOUND ( 'NONE', #14624, .T. ) ;
#2455=DIRECTION ( 'NONE',  ( -1.000000000000000000, 0.000000000000000000, 0.000000000000000000 ) ) ;
#2460=EDGE_LOOP ( 'NONE', ( #20784, #5794 ) ) ;
#2462=LINE ( 'NONE', #2258, #7559 ) ;
#2463=ORIENTED_EDGE ( 'NONE', *, *, #10375, .F. ) ;
#2465=CARTESIAN_POINT ( 'NONE',  ( 24.99999999999999289, -29.99999999999999645, -45.00000000000000000 ) ) ;
#2466=CARTESIAN_POINT ( 'NONE',  ( 0.000000000000000000, 0.000000000000000000, -81.99999999999998579 ) ) ;
#2472=EDGE_CURVE ( 'NONE', #14189, #4504, #8918, .T. ) ;
#2479=ADVANCED_FACE ( 'NONE', ( #4999 ), #11361, .T. ) ;
#2488=CARTESIAN_POINT ( 'NONE',  ( 30.00000000000000000, 4.299168419249259188, -84.99999999999998579 ) ) ;
#2489=VERTEX_POINT ( 'NONE', #8273 ) ;
#2491=CYLINDRICAL_SURFACE ( 'NONE', #13076, 63.70999227554992217 ) ;
#2495=AXIS2_PLACEMENT_3D ( 'NONE', #3186, #8365, #1613 ) ;
#2501=CARTESIAN_POINT ( 'NONE',  ( -30.00000000000000000, 36.35083268962915781, -50.00000000000000000 ) ) ;
#2504=ADVANCED_FACE ( 'NONE', ( #4895 ), #3308, .T. ) ;
#2516=CARTESIAN_POINT ( 'NONE',  ( -7.056982170014208577, -20.35833373244388511, 76.58484614278654590 ) ) ;
#2519=CYLINDRICAL_SURFACE ( 'NONE', #385, 5.000000000000000888 ) ;
#2523=CARTESIAN_POINT ( 'NONE',  ( -30.00000000000000000, -85.00000000000000000, -14.50000000000000533 ) ) ;
#2526=CARTESIAN_POINT ( 'NONE',  ( -9.591132434872761792, -20.91852224714069663, -76.31448437082826786 ) ) ;
#2528=DIRECTION ( 'NONE',  ( 0.6156453966108028641, 0.000000000000000000, 0.7880233154113698291 ) ) ;
#2531=ORIENTED_EDGE ( 'NONE', *, *, #4934, .T. ) ;
#2539=CARTESIAN_POINT ( 'NONE',  ( -8.500000000000000000, 1.040949779275250140E-15, 81.99999999999998579 ) ) ;
#2546=EDGE_LOOP ( 'NONE', ( #18740, #19824, #13697, #8968, #17911 ) ) ;
#2549=CARTESIAN_POINT ( 'NONE',  ( 30.00000000000000000, -122.0000000000000000, -6.368163355566234804E-15 ) ) ;
#2554=PLANE ( 'NONE',  #1595 ) ;
#2555=ORIENTED_EDGE ( 'NONE', *, *, #3243, .F. ) ;
#2556=VERTEX_POINT ( 'NONE', #12758 ) ;
#2560=PLANE ( 'NONE',  #9591 ) ;
#2561=EDGE_CURVE ( 'NONE', #11740, #6167, #4690, .T. ) ;
#2566=DIRECTION ( 'NONE',  ( 0.000000000000000000, 0.000000000000000000, 1.000000000000000000 ) ) ;
#2568=DIRECTION ( 'NONE',  ( 0.000000000000000000, 0.000000000000000000, 1.000000000000000000 ) ) ;
#2571=VECTOR ( 'NONE', #15402, 1000.000000000000000 ) ;
#2574=CARTESIAN_POINT ( 'NONE',  ( 0.6949845910673706495, -21.50225451306873481, 70.57937617215436887 ) ) ;
#2577=ORIENTED_EDGE ( 'NONE', *, *, #13101, .F. ) ;
#2579=CARTESIAN_POINT ( 'NONE',  ( 50.00000000000000000, -29.99999999999999645, -45.00000000000000000 ) ) ;
#2590=EDGE_LOOP ( 'NONE', ( #8518, #519, #2101, #6155, #17013 ) ) ;
#2591=AXIS2_PLACEMENT_3D ( 'NONE', #9741, #90, #6750 ) ;
#2594=EDGE_LOOP ( 'NONE', ( #3421, #12271 ) ) ;
#2595=CARTESIAN_POINT ( 'NONE',  ( -11.54691128655043642, -18.15138880902595275, -72.10074112616624120 ) ) ;
#2600=EDGE_CURVE ( 'NONE', #20455, #2408, #2333, .T. ) ;
#2604=LINE ( 'NONE', #4063, #19513 ) ;
#2608=VERTEX_POINT ( 'NONE', #3603 ) ;
#2609=CARTESIAN_POINT ( 'NONE',  ( 0.000000000000000000, 0.000000000000000000, 68.00000000000000000 ) ) ;
#2610=EDGE_CURVE ( 'NONE', #12500, #16359, #15355, .T. ) ;
#2621=VERTEX_POINT ( 'NONE', #15257 ) ;
#2622=CARTESIAN_POINT ( 'NONE',  ( -16.85739145898632074, -13.40013307497100925, 80.75697659352094604 ) ) ;
#2623=EDGE_CURVE ( 'NONE', #6843, #8495, #20078, .T. ) ;
#2624=AXIS2_PLACEMENT_3D ( 'NONE', #20264, #15399, #10130 ) ;
#2627=ADVANCED_FACE ( 'NONE', ( #13679 ), #13370, .F. ) ;
#2630=ORIENTED_EDGE ( 'NONE', *, *, #11328, .F. ) ;
#2636=CARTESIAN_POINT ( 'NONE',  ( 21.70015242457608196, -7.699555573020137267, -85.52161047917867620 ) ) ;
#2649=EDGE_CURVE ( 'NONE', #19553, #19211, #5300, .T. ) ;
#2662=ORIENTED_EDGE ( 'NONE', *, *, #19573, .T. ) ;
#2666=ORIENTED_EDGE ( 'NONE', *, *, #14193, .F. ) ;
#2667=CARTESIAN_POINT ( 'NONE',  ( 36.51810716189519468, -119.7975043377066697, -78.43191108116040766 ) ) ;
#2672=LINE ( 'NONE', #18989, #32 ) ;
#2673=DIRECTION ( 'NONE',  ( 0.000000000000000000, 1.000000000000000000, -8.673617379884034239E-17 ) ) ;
#2675=CYLINDRICAL_SURFACE ( 'NONE', #9198, 8.500000000000000000 ) ;
#2678=DIRECTION ( 'NONE',  ( -0.000000000000000000, -0.000000000000000000, -1.000000000000000000 ) ) ;
#2683=FACE_OUTER_BOUND ( 'NONE', #3001, .T. ) ;
#2686=ORIENTED_EDGE ( 'NONE', *, *, #12480, .F. ) ;
#2690=CARTESIAN_POINT ( 'NONE',  ( -30.00000000000000000, -170.8299878242309546, 15.48896927112552824 ) ) ;
#2695=CARTESIAN_POINT ( 'NONE',  ( 50.00000000000000000, -29.99999999999999645, -45.00000000000000000 ) ) ;
#2701=VERTEX_POINT ( 'NONE', #13476 ) ;
#2704=CARTESIAN_POINT ( 'NONE',  ( 50.00000000000000000, -164.9999999999999716, -90.00000000000001421 ) ) ;
#2706=ORIENTED_EDGE ( 'NONE', *, *, #18009, .T. ) ;
#2708=ADVANCED_FACE ( 'NONE', ( #10393 ), #8688, .T. ) ;
#2723=ORIENTED_EDGE ( 'NONE', *, *, #4912, .F. ) ;
#2724=CARTESIAN_POINT ( 'NONE',  ( -3.019303355814636269, -22.81398296884255927, -75.45291102792386084 ) ) ;
#2725=DIRECTION ( 'NONE',  ( -0.6156453966108041964, 0.000000000000000000, 0.7880233154113687188 ) ) ;
#2730=CARTESIAN_POINT ( 'NONE',  ( 30.00000000000000000, -99.99999999999998579, -52.00000000000000000 ) ) ;
#2739=EDGE_CURVE ( 'NONE', #13850, #1999, #15979, .T. ) ;
#2743=ORIENTED_EDGE ( 'NONE', *, *, #6389, .T. ) ;
#2747=VERTEX_POINT ( 'NONE', #5711 ) ;
#2753=DIRECTION ( 'NONE',  ( 1.000000000000000000, -0.000000000000000000, -0.000000000000000000 ) ) ;
#2754=AXIS2_PLACEMENT_3D ( 'NONE', #1842, #4914, #17858 ) ;
#2761=CARTESIAN_POINT ( 'NONE',  ( 37.15969169416875673, -120.3577465631687033, -78.81653076392491641 ) ) ;
#2766=DIRECTION ( 'NONE',  ( 1.000000000000000000, 0.000000000000000000, -0.000000000000000000 ) ) ;
#2784=CARTESIAN_POINT ( 'NONE',  ( 50.00000000000000000, -164.9999999999999716, 75.59990929030060158 ) ) ;
#2785=CYLINDRICAL_SURFACE ( 'NONE', #6653, 80.00000000000000000 ) ;
#2786=EDGE_LOOP ( 'NONE', ( #4513, #3181 ) ) ;
#2790=CARTESIAN_POINT ( 'NONE',  ( 24.99999999999999645, -39.99999999999999289, -52.00000000000000000 ) ) ;
#2794=ORIENTED_EDGE ( 'NONE', *, *, #8821, .T. ) ;
#2798=ORIENTED_EDGE ( 'NONE', *, *, #14879, .T. ) ;
#2799=VECTOR ( 'NONE', #19885, 1000.000000000000000 ) ;
#2805=VECTOR ( 'NONE', #6216, 1000.000000000000000 ) ;
#2812=ORIENTED_EDGE ( 'NONE', *, *, #7995, .F. ) ;
#2823=CARTESIAN_POINT ( 'NONE',  ( -1.464933908330800394, -21.46223383259977879, 76.05833375614351155 ) ) ;
#2832=ORIENTED_EDGE ( 'NONE', *, *, #3897, .F. ) ;
#2833=CARTESIAN_POINT ( 'NONE',  ( 19.24126430796853171, -12.61765026593414873, -81.34437286535597877 ) ) ;
#2852=EDGE_CURVE ( 'NONE', #11740, #5793, #1443, .T. ) ;
#2868=DIRECTION ( 'NONE',  ( -0.000000000000000000, -0.000000000000000000, 1.000000000000000000 ) ) ;
#2869=FACE_OUTER_BOUND ( 'NONE', #5666, .T. ) ;
#2877=CARTESIAN_POINT ( 'NONE',  ( 30.00000000000000000, -50.00000000000000000, -90.00000000000001421 ) ) ;
#2888=EDGE_LOOP ( 'NONE', ( #11612, #13345, #13289, #12087, #993, #4415, #17877, #15738, #10933, #2798, #11922, #17154, #17493, #858, #7916, #13524, #16055, #8102, #14543, #11910, #12792, #19990, #12548, #8448, #1874, #18556, #2338, #1405 ) ) ;
#2890=DIRECTION ( 'NONE',  ( 1.000000000000000000, 0.000000000000000000, -0.000000000000000000 ) ) ;
#2891=CARTESIAN_POINT ( 'NONE',  ( 0.000000000000000000, 0.000000000000000000, -84.99999999999998579 ) ) ;
#2894=CARTESIAN_POINT ( 'NONE',  ( 30.00000000000000711, -30.00000000000001421, -120.0000000000000142 ) ) ;
#2900=ORIENTED_EDGE ( 'NONE', *, *, #12503, .T. ) ;
#2901=ADVANCED_FACE ( 'NONE', ( #10715 ), #17179, .F. ) ;
#2906=ORIENTED_EDGE ( 'NONE', *, *, #11299, .T. ) ;
#2909=VECTOR ( 'NONE', #8162, 1000.000000000000000 ) ;
#2910=VERTEX_POINT ( 'NONE', #14723 ) ;
#2914=CARTESIAN_POINT ( 'NONE',  ( -30.00000000000000000, -30.00000000000000000, -130.0000000000000000 ) ) ;
#2923=AXIS2_PLACEMENT_3D ( 'NONE', #7245, #13727, #685 ) ;
#2932=DIRECTION ( 'NONE',  ( 1.000000000000000000, 0.000000000000000000, 0.000000000000000000 ) ) ;
#2936=CARTESIAN_POINT ( 'NONE',  ( -32.96694501150314949, -24.74873734152930993, -130.0000000000000000 ) ) ;
#2938=AXIS2_PLACEMENT_3D ( 'NONE', #594, #4180, #18602 ) ;
#2940=( GEOMETRIC_REPRESENTATION_CONTEXT ( 3 ) GLOBAL_UNCERTAINTY_ASSIGNED_CONTEXT ( ( #14939 ) ) GLOBAL_UNIT_ASSIGNED_CONTEXT ( ( #5009, #5206, #15169 ) ) REPRESENTATION_CONTEXT ( 'NONE', 'WORKASPACE' ) );
#2945=EDGE_CURVE ( 'NONE', #17868, #15579, #11337, .T. ) ;
#2957=CIRCLE ( 'NONE', #1932, 10.00000000000000178 ) ;
#2960=DIRECTION ( 'NONE',  ( -1.000000000000000000, 0.000000000000000000, 0.000000000000000000 ) ) ;
#2962=DIRECTION ( 'NONE',  ( 0.000000000000000000, 0.000000000000000000, -1.000000000000000000 ) ) ;
#2966=CARTESIAN_POINT ( 'NONE',  ( -24.99999999999999289, -85.00000000000000000, -9.000000000000005329 ) ) ;
#2969=DIRECTION ( 'NONE',  ( -1.000000000000000000, 0.000000000000000000, 0.000000000000000000 ) ) ;
#2977=ORIENTED_EDGE ( 'NONE', *, *, #5731, .F. ) ;
#2978=ORIENTED_EDGE ( 'NONE', *, *, #3510, .T. ) ;
#2994=CARTESIAN_POINT ( 'NONE',  ( 19.54001732319277096, -8.991134644608434812, 77.82005195698279465 ) ) ;
#2995=ORIENTED_EDGE ( 'NONE', *, *, #17866, .T. ) ;
#2996=CARTESIAN_POINT ( 'NONE',  ( 45.22159793441012710, -8.673994507468391291, -90.00000000000001421 ) ) ;
#3001=EDGE_LOOP ( 'NONE', ( #20430, #3753 ) ) ;
#3002=DIRECTION ( 'NONE',  ( 0.000000000000000000, 0.000000000000000000, -1.000000000000000000 ) ) ;
#3004=DIRECTION ( 'NONE',  ( -1.000000000000000000, 0.000000000000000000, 0.000000000000000000 ) ) ;
#3009=EDGE_CURVE ( 'NONE', #5467, #18936, #18006, .T. ) ;
#3012=EDGE_CURVE ( 'NONE', #10368, #12982, #16987, .T. ) ;
#3018=CARTESIAN_POINT ( 'NONE',  ( 10.00000000000000178, -160.0000000000000000, -70.00000000000000000 ) ) ;
#3019=B_SPLINE_CURVE_WITH_KNOTS ( 'NONE', 3,
 ( #3154, #1373, #7818, #20739 ),
 .UNSPECIFIED., .F., .F.,
 ( 4, 4 ),
 ( 0.000000000000000000, 0.005429897942433520482 ),
 .UNSPECIFIED. ) ;
#3024=ADVANCED_FACE ( 'NONE', ( #17702 ), #20865, .F. ) ;
#3027=DIRECTION ( 'NONE',  ( -1.000000000000000000, 0.000000000000000000, 0.000000000000000000 ) ) ;
#3035=ORIENTED_EDGE ( 'NONE', *, *, #1972, .F. ) ;
#3040=VECTOR ( 'NONE', #3239, 1000.000000000000000 ) ;
#3043=DIRECTION ( 'NONE',  ( -0.000000000000000000, -1.000000000000000000, -0.000000000000000000 ) ) ;
#3046=LINE ( 'NONE', #7810, #2805 ) ;
#3047=LINE ( 'NONE', #1472, #1224 ) ;
#3050=DIRECTION ( 'NONE',  ( -0.000000000000000000, -0.000000000000000000, 1.000000000000000000 ) ) ;
#3051=DIRECTION ( 'NONE',  ( 0.000000000000000000, 0.000000000000000000, -1.000000000000000000 ) ) ;
#3066=ORIENTED_EDGE ( 'NONE', *, *, #15195, .F. ) ;
#3071=ORIENTED_EDGE ( 'NONE', *, *, #9944, .F. ) ;
#3072=CARTESIAN_POINT ( 'NONE',  ( 50.00000000000000000, -164.9999999999999716, 90.00000000000001421 ) ) ;
#3083=FACE_OUTER_BOUND ( 'NONE', #3496, .T. ) ;
#3085=CARTESIAN_POINT ( 'NONE',  ( 0.000000000000000000, 0.000000000000000000, 81.99999999999998579 ) ) ;
#3086=EDGE_LOOP ( 'NONE', ( #914, #19433, #10017, #15743 ) ) ;
#3091=ORIENTED_EDGE ( 'NONE', *, *, #5199, .T. ) ;
#3093=DIRECTION ( 'NONE',  ( 0.000000000000000000, 0.000000000000000000, -1.000000000000000000 ) ) ;
#3096=CARTESIAN_POINT ( 'NONE',  ( 10.00000000000000178, -164.9999999999999716, 66.80000000000001137 ) ) ;
#3100=CYLINDRICAL_SURFACE ( 'NONE', #5265, 10.00000000000000178 ) ;
#3103=DIRECTION ( 'NONE',  ( 1.000000000000000000, -0.000000000000000000, -0.000000000000000000 ) ) ;
#3104=VECTOR ( 'NONE', #12705, 1000.000000000000000 ) ;
#3109=DIRECTION ( 'NONE',  ( -0.000000000000000000, -1.000000000000000000, -0.000000000000000000 ) ) ;
#3110=DIRECTION ( 'NONE',  ( 1.000000000000000000, -0.000000000000000000, -0.000000000000000000 ) ) ;
#3111=EDGE_LOOP ( 'NONE', ( #1091, #16142, #17240, #7839, #9407 ) ) ;
#3114=CARTESIAN_POINT ( 'NONE',  ( 0.000000000000000000, 0.000000000000000000, 68.00000000000000000 ) ) ;
#3123=ORIENTED_EDGE ( 'NONE', *, *, #11908, .T. ) ;
#3125=CARTESIAN_POINT ( 'NONE',  ( 50.00000000000000000, 31.35083268962919689, -84.99999999999998579 ) ) ;
#3129=CIRCLE ( 'NONE', #5830, 2.099999999999997868 ) ;
#3133=AXIS2_PLACEMENT_3D ( 'NONE', #20209, #6016, #5686 ) ;
#3134=ORIENTED_EDGE ( 'NONE', *, *, #13123, .T. ) ;
#3135=CARTESIAN_POINT ( 'NONE',  ( -0.7462824556787200914, -21.49896008043337403, 76.04131803729603689 ) ) ;
#3137=FACE_OUTER_BOUND ( 'NONE', #19583, .T. ) ;
#3147=CARTESIAN_POINT ( 'NONE',  ( 0.000000000000000000, 0.000000000000000000, 81.99999999999998579 ) ) ;
#3153=PLANE ( 'NONE',  #18184 ) ;
#3154=CARTESIAN_POINT ( 'NONE',  ( 43.62500077266425791, -125.0000000000000000, 90.00000000000002842 ) ) ;
#3159=DIRECTION ( 'NONE',  ( 1.000000000000000000, -0.000000000000000000, -0.000000000000000000 ) ) ;
#3166=DIRECTION ( 'NONE',  ( 0.000000000000000000, 1.000000000000000000, -3.469446951953615175E-16 ) ) ;
#3174=ORIENTED_EDGE ( 'NONE', *, *, #19914, .F. ) ;
#3176=DIRECTION ( 'NONE',  ( 1.000000000000000000, -0.000000000000000000, -0.000000000000000000 ) ) ;
#3178=CARTESIAN_POINT ( 'NONE',  ( 43.01509889268501752, -11.40594424968584519, -82.27917910797492596 ) ) ;
#3180=VERTEX_POINT ( 'NONE', #5789 ) ;
#3181=ORIENTED_EDGE ( 'NONE', *, *, #15051, .T. ) ;
#3184=EDGE_CURVE ( 'NONE', #4504, #19648, #4420, .T. ) ;
#3186=CARTESIAN_POINT ( 'NONE',  ( 30.00000000000000000, -85.00000000000000000, -1.040949779275250179E-14 ) ) ;
#3191=CARTESIAN_POINT ( 'NONE',  ( -32.96694501150314949, -24.74873734152930993, -120.0000000000000142 ) ) ;
#3192=CARTESIAN_POINT ( 'NONE',  ( 30.00000000000000000, -159.9999999999999716, 53.99496054166689873 ) ) ;
#3200=ORIENTED_EDGE ( 'NONE', *, *, #17105, .F. ) ;
#3202=EDGE_LOOP ( 'NONE', ( #18416, #16778, #6482, #10806 ) ) ;
#3206=VERTEX_POINT ( 'NONE', #17254 ) ;
#3207=CARTESIAN_POINT ( 'NONE',  ( 10.00000000000000178, -160.0000000000000000, 73.20000000000000284 ) ) ;
#3208=EDGE_CURVE ( 'NONE', #15761, #6177, #15544, .T. ) ;
#3213=PLANE ( 'NONE',  #9610 ) ;
#3226=ORIENTED_EDGE ( 'NONE', *, *, #19984, .T. ) ;
#3233=ADVANCED_FACE ( 'NONE', ( #20533 ), #17359, .T. ) ;
#3239=DIRECTION ( 'NONE',  ( -1.000000000000000000, 0.000000000000000000, 0.000000000000000000 ) ) ;
#3241=CYLINDRICAL_SURFACE ( 'NONE', #10061, 35.00000000000000000 ) ;
#3243=EDGE_CURVE ( 'NONE', #5413, #2556, #9980, .T. ) ;
#3249=AXIS2_PLACEMENT_3D ( 'NONE', #15106, #1865, #5247 ) ;
#3262=ADVANCED_FACE ( 'NONE', ( #1572 ), #14287, .T. ) ;
#3264=DIRECTION ( 'NONE',  ( 0.000000000000000000, 0.000000000000000000, -1.000000000000000000 ) ) ;
#3265=AXIS2_PLACEMENT_3D ( 'NONE', #7683, #15622, #9583 ) ;
#3270=ADVANCED_FACE ( 'NONE', ( #11413 ), #14595, .F. ) ;
#3275=LINE ( 'NONE', #3466, #18526 ) ;
#3276=ORIENTED_EDGE ( 'NONE', *, *, #7027, .F. ) ;
#3279=ORIENTED_EDGE ( 'NONE', *, *, #4958, .T. ) ;
#3284=EDGE_CURVE ( 'NONE', #2910, #19113, #11927, .T. ) ;
#3291=DIRECTION ( 'NONE',  ( -0.000000000000000000, -0.000000000000000000, 1.000000000000000000 ) ) ;
#3298=DIRECTION ( 'NONE',  ( -1.000000000000000000, -0.000000000000000000, -0.000000000000000000 ) ) ;
#3299=CARTESIAN_POINT ( 'NONE',  ( 50.00100000000000477, -85.00000000000000000, 8.999999999999984013 ) ) ;
#3306=DIRECTION ( 'NONE',  ( -1.000000000000000000, 0.000000000000000000, 0.000000000000000000 ) ) ;
#3308=PLANE ( 'NONE',  #5517 ) ;
#3314=ORIENTED_EDGE ( 'NONE', *, *, #10940, .T. ) ;
#3330=ORIENTED_EDGE ( 'NONE', *, *, #6200, .F. ) ;
#3331=DIRECTION ( 'NONE',  ( -1.000000000000000000, 0.000000000000000000, 0.000000000000000000 ) ) ;
#3336=CARTESIAN_POINT ( 'NONE',  ( 10.00000000000000178, -164.9999999999999716, -66.80000000000001137 ) ) ;
#3339=FACE_OUTER_BOUND ( 'NONE', #16825, .T. ) ;
#3342=CARTESIAN_POINT ( 'NONE',  ( -19.93133741578929730, -8.067442883292189393, -78.55234307929258364 ) ) ;
#3343=EDGE_CURVE ( 'NONE', #10522, #405, #3046, .T. ) ;
#3351=DIRECTION ( 'NONE',  ( 0.000000000000000000, 0.000000000000000000, 1.000000000000000000 ) ) ;
#3356=CARTESIAN_POINT ( 'NONE',  ( -30.00000000000000000, -85.00000000000000000, 11.49999999999998579 ) ) ;
#3361=DIRECTION ( 'NONE',  ( 0.000000000000000000, 0.000000000000000000, 1.000000000000000000 ) ) ;
#3366=CARTESIAN_POINT ( 'NONE',  ( 24.99999999999999289, -110.0000000000000142, 44.99999999999999289 ) ) ;
#3367=CARTESIAN_POINT ( 'NONE',  ( 43.03985923310276007, -11.23385978448955136, 76.06858800491698958 ) ) ;
#3368=EDGE_LOOP ( 'NONE', ( #1791, #9990, #13865, #20173, #2812, #9966 ) ) ;
#3369=EDGE_CURVE ( 'NONE', #13140, #11331, #10580, .T. ) ;
#3373=DIRECTION ( 'NONE',  ( 1.000000000000000000, 0.000000000000000000, 0.000000000000000000 ) ) ;
#3378=AXIS2_PLACEMENT_3D ( 'NONE', #10016, #5243, #8115 ) ;
#3380=ADVANCED_FACE ( 'NONE', ( #18395 ), #3864, .T. ) ;
#3382=CYLINDRICAL_SURFACE ( 'NONE', #5796, 20.00000000000000000 ) ;
#3386=LINE ( 'NONE', #3299, #3538 ) ;
#3387=LINE ( 'NONE', #11355, #4603 ) ;
#3393=DIRECTION ( 'NONE',  ( 0.000000000000000000, 0.000000000000000000, 1.000000000000000000 ) ) ;
#3394=VERTEX_POINT ( 'NONE', #11822 ) ;
#3395=EDGE_CURVE ( 'NONE', #18485, #4283, #6941, .T. ) ;
#3397=ORIENTED_EDGE ( 'NONE', *, *, #8433, .T. ) ;
#3398=DIRECTION ( 'NONE',  ( 0.000000000000000000, 0.000000000000000000, 1.000000000000000000 ) ) ;
#3404=EDGE_CURVE ( 'NONE', #14263, #1127, #17700, .T. ) ;
#3406=CARTESIAN_POINT ( 'NONE',  ( 30.00000000000000000, -99.99999999999998579, 52.00000000000000000 ) ) ;
#3414=DIRECTION ( 'NONE',  ( 1.000000000000000000, -1.734723475976806848E-16, -0.000000000000000000 ) ) ;
#3420=CARTESIAN_POINT ( 'NONE',  ( -40.00000000000000000, 29.99999999999999289, -130.0000000000000000 ) ) ;
#3421=ORIENTED_EDGE ( 'NONE', *, *, #17291, .T. ) ;
#3426=CIRCLE ( 'NONE', #19996, 8.999999999999994671 ) ;
#3427=AXIS2_PLACEMENT_3D ( 'NONE', #7740, #10717, #18773 ) ;
#3428=LINE ( 'NONE', #3125, #4328 ) ;
#3429=ADVANCED_FACE ( 'NONE', ( #6626 ), #6831, .F. ) ;
#3433=ORIENTED_EDGE ( 'NONE', *, *, #12990, .T. ) ;
#3436=VERTEX_POINT ( 'NONE', #10232 ) ;
#3443=CARTESIAN_POINT ( 'NONE',  ( 50.00000000000000000, -139.6410161513775563, -85.00000000000000000 ) ) ;
#3445=CARTESIAN_POINT ( 'NONE',  ( 28.13963350654227824, -26.35784117651622793, -120.0000000000000142 ) ) ;
#3447=CARTESIAN_POINT ( 'NONE',  ( 0.000000000000000000, 0.000000000000000000, -68.00000000000000000 ) ) ;
#3449=ORIENTED_EDGE ( 'NONE', *, *, #3404, .F. ) ;
#3450=DIRECTION ( 'NONE',  ( 0.000000000000000000, 0.000000000000000000, 1.000000000000000000 ) ) ;
#3452=CIRCLE ( 'NONE', #16317, 5.000000000000000888 ) ;
#3462=VECTOR ( 'NONE', #6084, 1000.000000000000000 ) ;
#3463=ORIENTED_EDGE ( 'NONE', *, *, #3654, .T. ) ;
#3466=CARTESIAN_POINT ( 'NONE',  ( -24.99999999999999289, 230.0000000000000000, -84.99999999999998579 ) ) ;
#3478=CIRCLE ( 'NONE', #14661, 5.000000000000004441 ) ;
#3496=EDGE_LOOP ( 'NONE', ( #6754, #7783, #1663, #2432 ) ) ;
#3499=CARTESIAN_POINT ( 'NONE',  ( 31.36240272394379858, -36.86890566740344610, -66.67347288640101510 ) ) ;
#3502=CARTESIAN_POINT ( 'NONE',  ( 50.00000000000000000, 36.35083268962915781, 50.00000000000000000 ) ) ;
#3505=AXIS2_PLACEMENT_3D ( 'NONE', #6432, #8235, #19577 ) ;
#3506=ADVANCED_FACE ( 'NONE', ( #5669 ), #13425, .T. ) ;
#3508=VECTOR ( 'NONE', #2241, 1000.000000000000000 ) ;
#3510=EDGE_CURVE ( 'NONE', #11331, #13140, #5162, .T. ) ;
#3513=CARTESIAN_POINT ( 'NONE',  ( 36.57435087158915366, -119.8477454916768181, -84.70193698065399701 ) ) ;
#3514=PLANE ( 'NONE',  #18968 ) ;
#3515=DIRECTION ( 'NONE',  ( 0.000000000000000000, 0.000000000000000000, -1.000000000000000000 ) ) ;
#3516=CARTESIAN_POINT ( 'NONE',  ( 29.74873734152916782, 24.74873734152916072, -120.0000000000000142 ) ) ;
#3520=ADVANCED_FACE ( 'NONE', ( #18608 ), #7254, .F. ) ;
#3526=VERTEX_POINT ( 'NONE', #2501 ) ;
#3527=DIRECTION ( 'NONE',  ( 1.000000000000000000, -0.000000000000000000, -0.000000000000000000 ) ) ;
#3530=AXIS2_PLACEMENT_3D ( 'NONE', #20236, #10173, #5604 ) ;
#3538=VECTOR ( 'NONE', #6460, 1000.000000000000000 ) ;
#3540=LINE ( 'NONE', #16682, #18987 ) ;
#3542=CARTESIAN_POINT ( 'NONE',  ( 10.00000000000000178, -160.0000000000000000, -66.80000000000001137 ) ) ;
#3557=PRODUCT_DEFINITION_SHAPE ( 'NONE', 'NONE',  #2358 ) ;
#3558=FACE_OUTER_BOUND ( 'NONE', #17089, .T. ) ;
#3561=ORIENTED_EDGE ( 'NONE', *, *, #5172, .T. ) ;
#3565=MANIFOLD_SOLID_BREP ( 'M6 Clearance Hole1', #17696 ) ;
#3566=AXIS2_PLACEMENT_3D ( 'NONE', #5910, #12381, #18849 ) ;
#3567=CARTESIAN_POINT ( 'NONE',  ( 30.00000000000000000, -85.00000000000000000, -1.040949779275250179E-14 ) ) ;
#3574=ORIENTED_EDGE ( 'NONE', *, *, #5563, .F. ) ;
#3577=PLANE ( 'NONE',  #20013 ) ;
#3578=DIRECTION ( 'NONE',  ( 1.000000000000000000, 0.000000000000000000, 0.000000000000000000 ) ) ;
#3583=VECTOR ( 'NONE', #4127, 1000.000000000000000 ) ;
#3592=CIRCLE ( 'NONE', #15799, 79.99999999999997158 ) ;
#3595=VECTOR ( 'NONE', #9362, 1000.000000000000000 ) ;
#3597=ADVANCED_FACE ( 'NONE', ( #19733 ), #3514, .T. ) ;
#3603=CARTESIAN_POINT ( 'NONE',  ( 30.00000000000000000, -49.99999999999999289, -71.93747284969079203 ) ) ;
#3609=DIRECTION ( 'NONE',  ( 0.000000000000000000, 0.000000000000000000, -1.000000000000000000 ) ) ;
#3613=CIRCLE ( 'NONE', #9389, 8.500000000000000000 ) ;
#3619=CARTESIAN_POINT ( 'NONE',  ( -25.00000000000000000, -30.00000000000000711, -58.09475019311124555 ) ) ;
#3623=VERTEX_POINT ( 'NONE', #5410 ) ;
#3626=CARTESIAN_POINT ( 'NONE',  ( 18.13963350654227469, -26.35784117651622793, -120.0000000000000142 ) ) ;
#3630=ORIENTED_EDGE ( 'NONE', *, *, #13538, .T. ) ;
#3637=CYLINDRICAL_SURFACE ( 'NONE', #18891, 2.099999999999997868 ) ;
#3640=DIRECTION ( 'NONE',  ( 1.000000000000000000, 0.000000000000000000, 0.000000000000000000 ) ) ;
#3646=FACE_OUTER_BOUND ( 'NONE', #6621, .T. ) ;
#3654=EDGE_CURVE ( 'NONE', #8524, #8783, #15987, .T. ) ;
#3656=ADVANCED_BREP_SHAPE_REPRESENTATION ( '', ( #3565, #12461 ), #2940 ) ;
#3659=CARTESIAN_POINT ( 'NONE',  ( 30.00000000000000000, -30.00000000000000711, 50.99019513592783426 ) ) ;
#3660=EDGE_CURVE ( 'NONE', #15594, #6600, #17381, .T. ) ;
#3662=CARTESIAN_POINT ( 'NONE',  ( 0.000000000000000000, 0.000000000000000000, -84.99999999999998579 ) ) ;
#3673=EDGE_CURVE ( 'NONE', #19655, #16611, #1491, .T. ) ;
#3675=CARTESIAN_POINT ( 'NONE',  ( 34.81051331576767183, -118.0383536556227995, 83.29664741859293997 ) ) ;
#3676=LINE ( 'NONE', #19679, #1283 ) ;
#3690=EDGE_CURVE ( 'NONE', #12734, #15337, #16967, .T. ) ;
#3694=CARTESIAN_POINT ( 'NONE',  ( -26.35784117651625280, 26.35784117651607872, -130.0000000000000000 ) ) ;
#3697=CARTESIAN_POINT ( 'NONE',  ( -24.99999999999999289, -159.9999999999999716, -85.00000000000000000 ) ) ;
#3706=ORIENTED_EDGE ( 'NONE', *, *, #9777, .T. ) ;
#3707=ORIENTED_EDGE ( 'NONE', *, *, #18942, .T. ) ;
#3710=EDGE_CURVE ( 'NONE', #20532, #3970, #15385, .T. ) ;
#3714=CARTESIAN_POINT ( 'NONE',  ( 31.32223236346404960, -112.1651446957970819, -79.86480430250811935 ) ) ;
#3724=CYLINDRICAL_SURFACE ( 'NONE', #106, 10.00000000000000178 ) ;
#3725=ORIENTED_EDGE ( 'NONE', *, *, #18967, .T. ) ;
#3730=AXIS2_PLACEMENT_3D ( 'NONE', #13514, #8414, #7237 ) ;
#3734=CARTESIAN_POINT ( 'NONE',  ( -23.00000000000000000, 2.816687638038912352E-15, -90.00000000000000000 ) ) ;
#3736=ORIENTED_EDGE ( 'NONE', *, *, #14493, .F. ) ;
#3738=DIRECTION ( 'NONE',  ( -1.000000000000000000, 0.000000000000000000, 0.000000000000000000 ) ) ;
#3740=CARTESIAN_POINT ( 'NONE',  ( 10.47959250967882738, -18.77674085041570606, -71.79709706900058563 ) ) ;
#3743=EDGE_CURVE ( 'NONE', #6167, #19712, #12539, .T. ) ;
#3745=CYLINDRICAL_SURFACE ( 'NONE', #4945, 5.000000000000004441 ) ;
#3747=EDGE_LOOP ( 'NONE', ( #14466, #12028, #9213, #18114, #14899, #13729, #2630 ) ) ;
#3753=ORIENTED_EDGE ( 'NONE', *, *, #12180, .F. ) ;
#3758=VECTOR ( 'NONE', #15586, 1000.000000000000000 ) ;
#3760=ORIENTED_EDGE ( 'NONE', *, *, #20339, .F. ) ;
#3771=CARTESIAN_POINT ( 'NONE',  ( 34.02361417125685250, -117.0388906796276700, 82.60709736717031149 ) ) ;
#3772=CARTESIAN_POINT ( 'NONE',  ( 50.00000000000000000, -139.6410161513775563, 85.00000000000000000 ) ) ;
#3774=AXIS2_PLACEMENT_3D ( 'NONE', #2609, #7140, #17010 ) ;
#3778=DIRECTION ( 'NONE',  ( -1.000000000000000000, 0.000000000000000000, 0.000000000000000000 ) ) ;
#3780=ORIENTED_EDGE ( 'NONE', *, *, #433, .T. ) ;
#3782=ORIENTED_EDGE ( 'NONE', *, *, #18434, .F. ) ;
#3783=CARTESIAN_POINT ( 'NONE',  ( -21.35784117651625280, 26.35784117651607872, -130.0000000000000000 ) ) ;
#3800=CARTESIAN_POINT ( 'NONE',  ( 0.000000000000000000, 0.000000000000000000, -130.0000000000000000 ) ) ;
#3803=CARTESIAN_POINT ( 'NONE',  ( -30.00000000000000000, -164.9999999999999716, 90.00000000000001421 ) ) ;
#3809=CARTESIAN_POINT ( 'NONE',  ( 50.00000000000000000, 36.35083268962920044, -90.00000000000000000 ) ) ;
#3811=( NAMED_UNIT ( * ) PLANE_ANGLE_UNIT ( ) SI_UNIT ( $, .RADIAN. ) );
#3813=FACE_OUTER_BOUND ( 'NONE', #8253, .T. ) ;
#3819=AXIS2_PLACEMENT_3D ( 'NONE', #582, #18592, #13927 ) ;
#3823=ORIENTED_EDGE ( 'NONE', *, *, #8501, .F. ) ;
#3827=CARTESIAN_POINT ( 'NONE',  ( -15.44968093174339963, -14.96845338175447360, 73.80849194119339529 ) ) ;
#3832=DIRECTION ( 'NONE',  ( 0.000000000000000000, 0.000000000000000000, 1.000000000000000000 ) ) ;
#3833=LINE ( 'NONE', #3939, #11727 ) ;
#3848=CYLINDRICAL_SURFACE ( 'NONE', #11531, 11.50000000000000000 ) ;
#3851=EDGE_CURVE ( 'NONE', #4973, #10522, #11796, .T. ) ;
#3852=CARTESIAN_POINT ( 'NONE',  ( 0.6949845910673885241, -21.50225451306873836, -70.57937617215435466 ) ) ;
#3858=EDGE_LOOP ( 'NONE', ( #15204, #4069, #7384, #9671 ) ) ;
#3861=AXIS2_PLACEMENT_3D ( 'NONE', #222, #20895, #12953 ) ;
#3864=PLANE ( 'NONE',  #1456 ) ;
#3881=ORIENTED_EDGE ( 'NONE', *, *, #3690, .T. ) ;
#3885=CARTESIAN_POINT ( 'NONE',  ( 24.99999999999999645, -39.99999999999999289, -49.89999999999999858 ) ) ;
#3887=EDGE_LOOP ( 'NONE', ( #7429, #8836, #13922 ) ) ;
#3888=ORIENTED_EDGE ( 'NONE', *, *, #6652, .T. ) ;
#3897=EDGE_CURVE ( 'NONE', #8714, #17156, #8152, .T. ) ;
#3900=CIRCLE ( 'NONE', #17469, 205.0000000000000284 ) ;
#3903=DIRECTION ( 'NONE',  ( -1.000000000000000000, 0.000000000000000000, 0.000000000000000000 ) ) ;
#3910=EDGE_CURVE ( 'NONE', #17156, #8714, #11201, .T. ) ;
#3911=DIRECTION ( 'NONE',  ( 0.000000000000000000, 0.000000000000000000, 1.000000000000000000 ) ) ;
#3914=CARTESIAN_POINT ( 'NONE',  ( -44.00000000000000000, -85.00000000000000000, -1.040949779275250179E-14 ) ) ;
#3926=DIRECTION ( 'NONE',  ( -1.000000000000000000, -0.000000000000000000, -0.000000000000000000 ) ) ;
#3929=AXIS2_PLACEMENT_3D ( 'NONE', #19561, #5037, #11500 ) ;
#3930=ORIENTED_EDGE ( 'NONE', *, *, #18063, .T. ) ;
#3938=CARTESIAN_POINT ( 'NONE',  ( 41.22647390543421864, -123.0286131151452196, 80.84140696824476890 ) ) ;
#3939=CARTESIAN_POINT ( 'NONE',  ( 50.00000000000000000, -105.0000000000000426, 77.45966692414833688 ) ) ;
#3943=AXIS2_PLACEMENT_3D ( 'NONE', #3662, #5256, #1981 ) ;
#3949=CIRCLE ( 'NONE', #7006, 5.000000000000004441 ) ;
#3953=DIRECTION ( 'NONE',  ( 1.000000000000000000, -0.000000000000000000, -0.000000000000000000 ) ) ;
#3957=AXIS2_PLACEMENT_3D ( 'NONE', #5817, #18649, #2969 ) ;
#3958=CARTESIAN_POINT ( 'NONE',  ( 14.87228507261737853, -15.53036221685706408, -73.48983352790762069 ) ) ;
#3960=AXIS2_PLACEMENT_3D ( 'NONE', #13193, #19641, #48 ) ;
#3963=CARTESIAN_POINT ( 'NONE',  ( 24.99999999999999645, -122.0000000000000000, 2.099999999999991207 ) ) ;
#3964=VERTEX_POINT ( 'NONE', #16165 ) ;
#3965=AXIS2_PLACEMENT_3D ( 'NONE', #7865, #12763, #2890 ) ;
#3970=VERTEX_POINT ( 'NONE', #19637 ) ;
#3974=CARTESIAN_POINT ( 'NONE',  ( 30.00000000000000000, -40.41646384503850697, -66.42520834682599684 ) ) ;
#3975=FACE_OUTER_BOUND ( 'NONE', #14612, .T. ) ;
#3981=ORIENTED_EDGE ( 'NONE', *, *, #3851, .T. ) ;
#3986=ORIENTED_EDGE ( 'NONE', *, *, #14658, .T. ) ;
#3987=CARTESIAN_POINT ( 'NONE',  ( 30.32166929073842709, -108.6878471672527269, 78.46984228986231358 ) ) ;
#3989=ORIENTED_EDGE ( 'NONE', *, *, #17647, .F. ) ;
#3990=CARTESIAN_POINT ( 'NONE',  ( -6.043644376632333781, -22.24467714164983079, -75.70091669079042163 ) ) ;
#3995=EDGE_LOOP ( 'NONE', ( #19762, #3330, #9556, #15232 ) ) ;
#3996=DIRECTION ( 'NONE',  ( 0.000000000000000000, -9.714451465470119729E-15, -1.000000000000000000 ) ) ;
#4006=EDGE_CURVE ( 'NONE', #231, #6577, #16940, .T. ) ;
#4007=ORIENTED_EDGE ( 'NONE', *, *, #6895, .F. ) ;
#4013=DIRECTION ( 'NONE',  ( 1.000000000000000000, 0.000000000000000000, 0.000000000000000000 ) ) ;
#4015=CARTESIAN_POINT ( 'NONE',  ( -24.99999999999999289, -1.326995226329896749, 84.99999999999998579 ) ) ;
#4017=EDGE_CURVE ( 'NONE', #20752, #13475, #15503, .T. ) ;
#4020=EDGE_LOOP ( 'NONE', ( #17875, #1699, #5148, #10890, #3930, #12692 ) ) ;
#4022=VECTOR ( 'NONE', #16126, 1000.000000000000000 ) ;
#4025=CARTESIAN_POINT ( 'NONE',  ( 10.00000000000000178, -164.9999999999999716, -70.00000000000000000 ) ) ;
#4027=EDGE_CURVE ( 'NONE', #10832, #7909, #15086, .T. ) ;
#4032=CARTESIAN_POINT ( 'NONE',  ( 50.00000000000000000, 230.0000000000000000, 0.000000000000000000 ) ) ;
#4033=EDGE_CURVE ( 'NONE', #5350, #1631, #944, .T. ) ;
#4040=CARTESIAN_POINT ( 'NONE',  ( 5.982253535725046589, -20.70709046307244350, 70.91533586927069166 ) ) ;
#4041=VERTEX_POINT ( 'NONE', #4155 ) ;
#4042=CARTESIAN_POINT ( 'NONE',  ( 30.00000000000000000, -30.00000000000000711, 58.09475019311124555 ) ) ;
#4043=ORIENTED_EDGE ( 'NONE', *, *, #8330, .F. ) ;
#4046=FACE_OUTER_BOUND ( 'NONE', #5304, .T. ) ;
#4063=CARTESIAN_POINT ( 'NONE',  ( 50.00000000000000000, -1.326995226329893862, 84.99999999999998579 ) ) ;
#4066=EDGE_LOOP ( 'NONE', ( #15507, #11578, #6536, #20580 ) ) ;
#4069=ORIENTED_EDGE ( 'NONE', *, *, #12570, .T. ) ;
#4070=DIRECTION ( 'NONE',  ( 0.000000000000000000, 0.000000000000000000, 1.000000000000000000 ) ) ;
#4072=AXIS2_PLACEMENT_3D ( 'NONE', #17732, #8083, #3398 ) ;
#4075=CYLINDRICAL_SURFACE ( 'NONE', #14992, 5.000000000000004441 ) ;
#4079=CARTESIAN_POINT ( 'NONE',  ( 24.74873734152916072, 24.74873734152916072, -130.0000000000000000 ) ) ;
#4081=CARTESIAN_POINT ( 'NONE',  ( -21.18805271706017379, -3.649167310370820871, 90.00000000000000000 ) ) ;
#4089=CARTESIAN_POINT ( 'NONE',  ( 16.72766586881387951, -15.78946417207352226, -79.16083386016902068 ) ) ;
#4093=EDGE_CURVE ( 'NONE', #14747, #10832, #17096, .T. ) ;
#4096=DIRECTION ( 'NONE',  ( -0.000000000000000000, -1.000000000000000000, -0.000000000000000000 ) ) ;
#4099=FACE_BOUND ( 'NONE', #8086, .T. ) ;
#4100=DIRECTION ( 'NONE',  ( 0.000000000000000000, 0.000000000000000000, -1.000000000000000000 ) ) ;
#4114=AXIS2_PLACEMENT_3D ( 'NONE', #1940, #8803, #5220 ) ;
#4123=CARTESIAN_POINT ( 'NONE',  ( 30.00000000000000000, -39.99999999999999289, 52.00000000000000000 ) ) ;
#4127=DIRECTION ( 'NONE',  ( -1.000000000000000000, 0.000000000000000000, 0.000000000000000000 ) ) ;
#4128=FACE_OUTER_BOUND ( 'NONE', #4604, .T. ) ;
#4133=CARTESIAN_POINT ( 'NONE',  ( -25.00000000000000000, -30.00000000000000711, 58.09475019311124555 ) ) ;
#4134=AXIS2_PLACEMENT_3D ( 'NONE', #4944, #4529, #3351 ) ;
#4137=CARTESIAN_POINT ( 'NONE',  ( -24.99999999999999289, 230.0000000000000000, -85.00000000000000000 ) ) ;
#4138=EDGE_CURVE ( 'NONE', #17904, #1745, #14593, .T. ) ;
#4139=CARTESIAN_POINT ( 'NONE',  ( -21.50000000000000000, 2.632990618166809235E-15, 68.00000000000000000 ) ) ;
#4148=CARTESIAN_POINT ( 'NONE',  ( -19.93133741578929730, -8.067442883292187616, 78.55234307929261206 ) ) ;
#4155=CARTESIAN_POINT ( 'NONE',  ( 30.00000000000000000, -148.4917293642369884, -48.67032260359990659 ) ) ;
#4158=VERTEX_POINT ( 'NONE', #18474 ) ;
#4159=CARTESIAN_POINT ( 'NONE',  ( -26.35784117651625280, 26.35784117651607872, -120.0000000000000142 ) ) ;
#4161=VECTOR ( 'NONE', #15732, 1000.000000000000000 ) ;
#4162=DIRECTION ( 'NONE',  ( 1.000000000000000000, 0.000000000000000000, 0.000000000000000000 ) ) ;
#4168=CARTESIAN_POINT ( 'NONE',  ( 25.00000000000000000, -30.00000000000000711, -50.99019513592786268 ) ) ;
#4176=CARTESIAN_POINT ( 'NONE',  ( 11.44271251907791687, -18.21718295280815880, -72.06823551977505815 ) ) ;
#4179=CYLINDRICAL_SURFACE ( 'NONE', #16838, 10.00000000000000178 ) ;
#4180=DIRECTION ( 'NONE',  ( 0.000000000000000000, 0.000000000000000000, 1.000000000000000000 ) ) ;
#4181=CIRCLE ( 'NONE', #8931, 5.000000000000004441 ) ;
#4184=VECTOR ( 'NONE', #17323, 1000.000000000000000 ) ;
#4186=VERTEX_POINT ( 'NONE', #14135 ) ;
#4187=CYLINDRICAL_SURFACE ( 'NONE', #3774, 11.50000000000000000 ) ;
#4199=ORIENTED_EDGE ( 'NONE', *, *, #6272, .T. ) ;
#4210=VECTOR ( 'NONE', #11263, 1000.000000000000000 ) ;
#4212=CARTESIAN_POINT ( 'NONE',  ( 22.55358526068749114, -4.614239574836358493, -88.80301248374354373 ) ) ;
#4218=CARTESIAN_POINT ( 'NONE',  ( -44.00000000000000000, -85.00000000000000000, -1.040949779275250179E-14 ) ) ;
#4226=ORIENTED_EDGE ( 'NONE', *, *, #7570, .F. ) ;
#4231=DIRECTION ( 'NONE',  ( -1.000000000000000000, 0.000000000000000000, 0.000000000000000000 ) ) ;
#4232=VECTOR ( 'NONE', #13666, 1000.000000000000000 ) ;
#4236=DIRECTION ( 'NONE',  ( 0.000000000000000000, 0.000000000000000000, -1.000000000000000000 ) ) ;
#4242=ORIENTED_EDGE ( 'NONE', *, *, #18942, .F. ) ;
#4244=PRODUCT_DEFINITION_FORMATION_WITH_SPECIFIED_SOURCE ( 'ANY', '', #7468, .NOT_KNOWN. ) ;
#4247=FACE_BOUND ( 'NONE', #19517, .T. ) ;
#4254=PLANE ( 'NONE',  #1885 ) ;
#4256=DIRECTION ( 'NONE',  ( 1.000000000000000000, 0.000000000000000000, 0.000000000000000000 ) ) ;
#4260=CARTESIAN_POINT ( 'NONE',  ( 17.61872475889258993, -12.39310755016576948, 75.38263485905284256 ) ) ;
#4275=EDGE_CURVE ( 'NONE', #14705, #6265, #15818, .T. ) ;
#4276=AXIS2_PLACEMENT_3D ( 'NONE', #13169, #1638, #3609 ) ;
#4283=VERTEX_POINT ( 'NONE', #11052 ) ;
#4291=ORIENTED_EDGE ( 'NONE', *, *, #12075, .F. ) ;
#4294=CIRCLE ( 'NONE', #4972, 40.00000000000000000 ) ;
#4300=CIRCLE ( 'NONE', #8689, 18.00000000000000000 ) ;
#4301=ADVANCED_FACE ( 'NONE', ( #2024 ), #19514, .T. ) ;
#4302=EDGE_CURVE ( 'NONE', #2621, #12626, #15931, .T. ) ;
#4303=CARTESIAN_POINT ( 'NONE',  ( 31.43473485066228079, -112.4512879816791013, 74.54413784199456927 ) ) ;
#4305=DIRECTION ( 'NONE',  ( 0.000000000000000000, 0.000000000000000000, -1.000000000000000000 ) ) ;
#4308=ORIENTED_EDGE ( 'NONE', *, *, #4497, .F. ) ;
#4309=VECTOR ( 'NONE', #13528, 1000.000000000000000 ) ;
#4311=ORIENTED_EDGE ( 'NONE', *, *, #6011, .F. ) ;
#4312=DIRECTION ( 'NONE',  ( 0.000000000000000000, 0.000000000000000000, 1.000000000000000000 ) ) ;
#4324=CARTESIAN_POINT ( 'NONE',  ( 10.68115262102694807, -20.37288806868372149, -76.58146718639416406 ) ) ;
#4325=LINE ( 'NONE', #17255, #12391 ) ;
#4328=VECTOR ( 'NONE', #9898, 1000.000000000000000 ) ;
#4334=CARTESIAN_POINT ( 'NONE',  ( 23.13963350654227824, -26.35784117651622793, -120.0000000000000142 ) ) ;
#4345=CARTESIAN_POINT ( 'NONE',  ( 24.99999999999999645, -99.99999999999998579, -52.00000000000000000 ) ) ;
#4348=ORIENTED_EDGE ( 'NONE', *, *, #2365, .F. ) ;
#4354=ORIENTED_EDGE ( 'NONE', *, *, #13484, .T. ) ;
#4359=CARTESIAN_POINT ( 'NONE',  ( 50.00000000000000000, -124.9999999999999858, 90.00000000000001421 ) ) ;
#4365=FACE_OUTER_BOUND ( 'NONE', #19281, .T. ) ;
#4369=ORIENTED_EDGE ( 'NONE', *, *, #5087, .F. ) ;
#4376=DIRECTION ( 'NONE',  ( 1.000000000000000000, 0.000000000000000000, 0.000000000000000000 ) ) ;
#4381=FACE_OUTER_BOUND ( 'NONE', #14061, .T. ) ;
#4387=LINE ( 'NONE', #17438, #14334 ) ;
#4392=SHAPE_REPRESENTATION ( 'Sealed Cast Iron Gearbox Casing', ( #12461 ), #2940 ) ;
#4395=ORIENTED_EDGE ( 'NONE', *, *, #1946, .T. ) ;
#4397=ORIENTED_EDGE ( 'NONE', *, *, #10568, .F. ) ;
#4398=VECTOR ( 'NONE', #9473, 1000.000000000000000 ) ;
#4401=DIRECTION ( 'NONE',  ( 0.000000000000000000, 0.000000000000000000, -1.000000000000000000 ) ) ;
#4407=CARTESIAN_POINT ( 'NONE',  ( -30.00000000000000000, -151.4095880458873467, 44.60680010464249534 ) ) ;
#4408=ORIENTED_EDGE ( 'NONE', *, *, #5089, .T. ) ;
#4409=CARTESIAN_POINT ( 'NONE',  ( -3.612956115288154635, -21.20621163160360112, 76.17826316794804598 ) ) ;
#4415=ORIENTED_EDGE ( 'NONE', *, *, #11009, .T. ) ;
#4416=CARTESIAN_POINT ( 'NONE',  ( -24.99999999999999289, -113.2094389508847314, 74.86138894033631175 ) ) ;
#4417=CYLINDRICAL_SURFACE ( 'NONE', #17190, 3.199999999999994404 ) ;
#4418=VECTOR ( 'NONE', #11120, 1000.000000000000000 ) ;
#4420=LINE ( 'NONE', #7383, #15658 ) ;
#4439=EDGE_CURVE ( 'NONE', #16465, #7909, #10082, .T. ) ;
#4447=CARTESIAN_POINT ( 'NONE',  ( 40.91005719111474548, -14.31667062835577120, -80.10683058186114636 ) ) ;
#4450=CIRCLE ( 'NONE', #17317, 2.099999999999990763 ) ;
#4459=AXIS2_PLACEMENT_3D ( 'NONE', #17643, #6396, #6294 ) ;
#4462=VECTOR ( 'NONE', #1698, 1000.000000000000000 ) ;
#4469=CYLINDRICAL_SURFACE ( 'NONE', #9959, 55.00000000000000711 ) ;
#4473=ORIENTED_EDGE ( 'NONE', *, *, #14171, .F. ) ;
#4479=VECTOR ( 'NONE', #8564, 1000.000000000000000 ) ;
#4482=VECTOR ( 'NONE', #8248, 1000.000000000000000 ) ;
#4483=DIRECTION ( 'NONE',  ( 1.000000000000000000, -1.387778780781445676E-15, 0.000000000000000000 ) ) ;
#4485=DIRECTION ( 'NONE',  ( 1.000000000000000000, 0.000000000000000000, 0.000000000000000000 ) ) ;
#4487=VERTEX_POINT ( 'NONE', #2335 ) ;
#4492=DIRECTION ( 'NONE',  ( -1.000000000000000000, 0.000000000000000000, 0.000000000000000000 ) ) ;
#4497=EDGE_CURVE ( 'NONE', #17002, #19648, #4450, .T. ) ;
#4504=VERTEX_POINT ( 'NONE', #15061 ) ;
#4513=ORIENTED_EDGE ( 'NONE', *, *, #3743, .T. ) ;
#4518=AXIS2_PLACEMENT_3D ( 'NONE', #8355, #3578, #11445 ) ;
#4519=CARTESIAN_POINT ( 'NONE',  ( 11.40258492152624115, -18.23049771964689825, 77.70848679321215968 ) ) ;
#4526=DIRECTION ( 'NONE',  ( 1.000000000000000000, 0.000000000000000000, 0.000000000000000000 ) ) ;
#4527=ORIENTED_EDGE ( 'NONE', *, *, #12542, .F. ) ;
#4529=DIRECTION ( 'NONE',  ( -1.000000000000000000, -0.000000000000000000, -0.000000000000000000 ) ) ;
#4530=DIRECTION ( 'NONE',  ( 0.000000000000000000, 0.000000000000000000, -1.000000000000000000 ) ) ;
#4536=FACE_BOUND ( 'NONE', #12063, .T. ) ;
#4537=CARTESIAN_POINT ( 'NONE',  ( -30.00000000000000000, -85.00000000000000000, -1.040949779275250179E-14 ) ) ;
#4549=CARTESIAN_POINT ( 'NONE',  ( 18.13963350654227469, -26.35784117651622793, -120.0000000000000142 ) ) ;
#4564=ORIENTED_EDGE ( 'NONE', *, *, #12360, .T. ) ;
#4565=CARTESIAN_POINT ( 'NONE',  ( 31.43268490318742181, -112.4462444941460006, -74.54209189151036696 ) ) ;
#4566=ADVANCED_FACE ( 'NONE', ( #19821 ), #642, .T. ) ;
#4568=DIRECTION ( 'NONE',  ( 0.000000000000000000, 0.000000000000000000, -1.000000000000000000 ) ) ;
#4569=FACE_OUTER_BOUND ( 'NONE', #20072, .T. ) ;
#4574=ADVANCED_FACE ( 'NONE', ( #11774, #13682 ), #18239, .T. ) ;
#4582=DIRECTION ( 'NONE',  ( 0.000000000000000000, -0.000000000000000000, 1.000000000000000000 ) ) ;
#4597=VERTEX_POINT ( 'NONE', #4015 ) ;
#4600=ORIENTED_EDGE ( 'NONE', *, *, #2739, .T. ) ;
#4602=CARTESIAN_POINT ( 'NONE',  ( 30.00000000000000000, -42.57363661491096707, 121.3828884801879155 ) ) ;
#4603=VECTOR ( 'NONE', #6368, 1000.000000000000000 ) ;
#4604=EDGE_LOOP ( 'NONE', ( #7890, #11418, #6378, #6773, #8023 ) ) ;
#4607=DIRECTION ( 'NONE',  ( 1.000000000000000000, -0.000000000000000000, -0.000000000000000000 ) ) ;
#4624=CARTESIAN_POINT ( 'NONE',  ( 21.03310778584661023, -4.548819502657031499, 88.88415356777898069 ) ) ;
#4626=AXIS2_PLACEMENT_3D ( 'NONE', #7815, #14086, #20538 ) ;
#4632=( GEOMETRIC_REPRESENTATION_CONTEXT ( 3 ) GLOBAL_UNCERTAINTY_ASSIGNED_CONTEXT ( ( #12390 ) ) GLOBAL_UNIT_ASSIGNED_CONTEXT ( ( #1927, #3811, #10297 ) ) REPRESENTATION_CONTEXT ( 'NONE', 'WORKASPACE' ) );
#4634=DIRECTION ( 'NONE',  ( 1.000000000000000000, 0.000000000000000000, -0.000000000000000000 ) ) ;
#4635=ORIENTED_EDGE ( 'NONE', *, *, #5169, .F. ) ;
#4636=CARTESIAN_POINT ( 'NONE',  ( -21.68676924570646847, -7.739453413396359061, -85.48199181195725771 ) ) ;
#4644=DIRECTION ( 'NONE',  ( -1.000000000000000000, 0.000000000000000000, 0.000000000000000000 ) ) ;
#4649=AXIS2_PLACEMENT_3D ( 'NONE', #3694, #15049, #3903 ) ;
#4651=ORIENTED_EDGE ( 'NONE', *, *, #2610, .F. ) ;
#4653=DIRECTION ( 'NONE',  ( -1.000000000000000000, 0.000000000000000000, 0.000000000000000000 ) ) ;
#4663=CARTESIAN_POINT ( 'NONE',  ( 29.99999999999999289, -49.01438689058709741, 66.75225413593169321 ) ) ;
#4667=ORIENTED_EDGE ( 'NONE', *, *, #14660, .T. ) ;
#4668=CARTESIAN_POINT ( 'NONE',  ( -24.99999999999999289, -85.00000000000000000, -1.040949779275250179E-14 ) ) ;
#4672=CARTESIAN_POINT ( 'NONE',  ( 32.33881229855617789, -114.4241705253154606, -75.39503781669127136 ) ) ;
#4674=AXIS2_PLACEMENT_3D ( 'NONE', #2790, #4162, #17102 ) ;
#4677=EDGE_CURVE ( 'NONE', #9768, #2130, #18319, .T. ) ;
#4679=EDGE_CURVE ( 'NONE', #16876, #9376, #1410, .T. ) ;
#4680=CARTESIAN_POINT ( 'NONE',  ( 30.00000000000000000, -42.57363661491096707, -121.3828884801879155 ) ) ;
#4685=VERTEX_POINT ( 'NONE', #6139 ) ;
#4690=LINE ( 'NONE', #11150, #15701 ) ;
#4693=DIRECTION ( 'NONE',  ( 0.000000000000000000, 0.000000000000000000, -1.000000000000000000 ) ) ;
#4699=EDGE_CURVE ( 'NONE', #5439, #14211, #8485, .T. ) ;
#4700=DIRECTION ( 'NONE',  ( -1.000000000000000000, 1.734723475976807094E-16, 0.000000000000000000 ) ) ;
#4707=DIRECTION ( 'NONE',  ( 0.000000000000000000, 0.000000000000000000, -1.000000000000000000 ) ) ;
#4711=CARTESIAN_POINT ( 'NONE',  ( 0.000000000000000000, 0.000000000000000000, 90.00000000000000000 ) ) ;
#4712=DIRECTION ( 'NONE',  ( -1.000000000000000000, -0.000000000000000000, -0.000000000000000000 ) ) ;
#4724=CARTESIAN_POINT ( 'NONE',  ( 40.00000000000000711, -40.00000000000001421, -120.0000000000000142 ) ) ;
#4727=VERTEX_POINT ( 'NONE', #20761 ) ;
#4728=CARTESIAN_POINT ( 'NONE',  ( 19.08980715481771995, -9.906743869288808568, 83.52356801772648964 ) ) ;
#4735=CARTESIAN_POINT ( 'NONE',  ( -30.00000000000000000, -105.0000000000000284, -77.45966692414833688 ) ) ;
#4738=CARTESIAN_POINT ( 'NONE',  ( 0.000000000000000000, 0.000000000000000000, -130.0000000000000000 ) ) ;
#4747=CARTESIAN_POINT ( 'NONE',  ( 50.00000000000000000, -139.6410161513775563, -90.00000000000001421 ) ) ;
#4751=EDGE_CURVE ( 'NONE', #20537, #20612, #12359, .T. ) ;
#4756=CARTESIAN_POINT ( 'NONE',  ( 31.45428956093201123, -36.32466546818508135, 66.70503744075557506 ) ) ;
#4759=ORIENTED_EDGE ( 'NONE', *, *, #5809, .F. ) ;
#4762=VECTOR ( 'NONE', #9030, 1000.000000000000000 ) ;
#4765=CARTESIAN_POINT ( 'NONE',  ( 47.39552796998189166, -5.594374250344187338, 80.66125912922146313 ) ) ;
#4766=VECTOR ( 'NONE', #2246, 1000.000000000000000 ) ;
#4767=AXIS2_PLACEMENT_3D ( 'NONE', #11893, #3832, #13819 ) ;
#4783=VERTEX_POINT ( 'NONE', #1501 ) ;
#4791=EDGE_CURVE ( 'NONE', #6575, #9434, #16308, .T. ) ;
#4795=CIRCLE ( 'NONE', #11601, 49.99999999999998579 ) ;
#4800=ORIENTED_EDGE ( 'NONE', *, *, #2365, .T. ) ;
#4804=CARTESIAN_POINT ( 'NONE',  ( 50.00000000000000000, 4.299168419249259188, -90.00000000000000000 ) ) ;
#4807=DIRECTION ( 'NONE',  ( 0.000000000000000000, 0.000000000000000000, 1.000000000000000000 ) ) ;
#4809=LINE ( 'NONE', #11277, #20091 ) ;
#4815=LINE ( 'NONE', #17559, #15975 ) ;
#4819=DIRECTION ( 'NONE',  ( -0.000000000000000000, -0.000000000000000000, -1.000000000000000000 ) ) ;
#4821=LINE ( 'NONE', #11290, #8222 ) ;
#4826=PLANE ( 'NONE',  #6584 ) ;
#4827=AXIS2_PLACEMENT_3D ( 'NONE', #6744, #3166, #10047 ) ;
#4831=CARTESIAN_POINT ( 'NONE',  ( 11.69263306866421814, -18.04574728598160505, 77.81190555643075868 ) ) ;
#4833=FACE_OUTER_BOUND ( 'NONE', #16559, .T. ) ;
#4835=EDGE_CURVE ( 'NONE', #9196, #5499, #9533, .T. ) ;
#4837=ORIENTED_EDGE ( 'NONE', *, *, #12432, .F. ) ;
#4843=CYLINDRICAL_SURFACE ( 'NONE', #11026, 200.0000000000000000 ) ;
#4845=ADVANCED_FACE ( 'NONE', ( #9649, #18110, #11340, #13143, #7950, #8057 ), #3577, .F. ) ;
#4846=ORIENTED_EDGE ( 'NONE', *, *, #5155, .T. ) ;
#4866=CIRCLE ( 'NONE', #16039, 23.00000000000000000 ) ;
#4868=AXIS2_PLACEMENT_3D ( 'NONE', #2695, #12668, #16048 ) ;
#4873=ORIENTED_EDGE ( 'NONE', *, *, #572, .F. ) ;
#4880=EDGE_CURVE ( 'NONE', #13026, #11744, #12932, .T. ) ;
#4881=CARTESIAN_POINT ( 'NONE',  ( 50.00000000000000000, -110.0000000000000142, 44.99999999999999289 ) ) ;
#4883=VECTOR ( 'NONE', #17104, 1000.000000000000000 ) ;
#4893=PLANE ( 'NONE',  #6570 ) ;
#4895=FACE_OUTER_BOUND ( 'NONE', #9617, .T. ) ;
#4900=ORIENTED_EDGE ( 'NONE', *, *, #2945, .T. ) ;
#4904=ADVANCED_FACE ( 'NONE', ( #95 ), #13034, .T. ) ;
#4912=EDGE_CURVE ( 'NONE', #10368, #12559, #11528, .T. ) ;
#4913=ORIENTED_EDGE ( 'NONE', *, *, #7784, .F. ) ;
#4914=DIRECTION ( 'NONE',  ( -0.000000000000000000, -0.000000000000000000, 1.000000000000000000 ) ) ;
#4923=CARTESIAN_POINT ( 'NONE',  ( 39.24629858617094413, -121.8853583615259311, 79.93655681056323203 ) ) ;
#4927=ORIENTED_EDGE ( 'NONE', *, *, #2081, .F. ) ;
#4931=VERTEX_POINT ( 'NONE', #11747 ) ;
#4934=EDGE_CURVE ( 'NONE', #19113, #2910, #18335, .T. ) ;
#4938=VERTEX_POINT ( 'NONE', #3885 ) ;
#4944=CARTESIAN_POINT ( 'NONE',  ( 50.00100000000000477, -85.00000000000000000, -1.040949779275250179E-14 ) ) ;
#4945=AXIS2_PLACEMENT_3D ( 'NONE', #5036, #8520, #19873 ) ;
#4947=DIRECTION ( 'NONE',  ( 1.000000000000000000, 0.000000000000000000, 0.000000000000000000 ) ) ;
#4958=EDGE_CURVE ( 'NONE', #20612, #16461, #8764, .T. ) ;
#4963=CARTESIAN_POINT ( 'NONE',  ( 0.000000000000000000, 0.000000000000000000, -68.00000000000000000 ) ) ;
#4972=AXIS2_PLACEMENT_3D ( 'NONE', #19997, #18430, #8770 ) ;
#4973=VERTEX_POINT ( 'NONE', #18423 ) ;
#4974=CARTESIAN_POINT ( 'NONE',  ( 30.00000000000000000, -85.00000000000000000, -1.040949779275250179E-14 ) ) ;
#4975=CARTESIAN_POINT ( 'NONE',  ( 24.99999999999999645, -39.99999999999999289, 54.09999999999999432 ) ) ;
#4976=CIRCLE ( 'NONE', #591, 35.00000000000001421 ) ;
#4977=ORIENTED_EDGE ( 'NONE', *, *, #6647, .T. ) ;
#4979=CARTESIAN_POINT ( 'NONE',  ( 46.24771825328784303, -7.470032835629814016, -79.01456834021801967 ) ) ;
#4980=VECTOR ( 'NONE', #18845, 1000.000000000000000 ) ;
#4990=AXIS2_PLACEMENT_3D ( 'NONE', #17891, #8228, #13213 ) ;
#4997=CARTESIAN_POINT ( 'NONE',  ( 10.00000000000000178, -40.41646384503856382, 66.42520834682601105 ) ) ;
#4999=FACE_OUTER_BOUND ( 'NONE', #15942, .T. ) ;
#5000=EDGE_LOOP ( 'NONE', ( #15911, #11132, #20497, #11180 ) ) ;
#5002=CARTESIAN_POINT ( 'NONE',  ( 32.12996668197559558, -33.64348109762138961, -67.10678061411157103 ) ) ;
#5007=CARTESIAN_POINT ( 'NONE',  ( 30.00000000000000000, -105.0000000000000000, -72.35596062816881613 ) ) ;
#5009=( LENGTH_UNIT ( ) NAMED_UNIT ( * ) SI_UNIT ( .MILLI., .METRE. ) );
#5010=LINE ( 'NONE', #14755, #6912 ) ;
#5018=DIRECTION ( 'NONE',  ( -1.000000000000000000, -0.000000000000000000, -0.000000000000000000 ) ) ;
#5023=LINE ( 'NONE', #9586, #19408 ) ;
#5034=CARTESIAN_POINT ( 'NONE',  ( 50.00000000000000000, 4.299168419249266293, 84.99999999999998579 ) ) ;
#5036=CARTESIAN_POINT ( 'NONE',  ( 24.74873734152916072, 24.74873734152916072, -120.0000000000000142 ) ) ;
#5037=DIRECTION ( 'NONE',  ( 0.000000000000000000, 0.000000000000000000, -1.000000000000000000 ) ) ;
#5042=DIRECTION ( 'NONE',  ( 0.000000000000000000, 0.000000000000000000, -1.000000000000000000 ) ) ;
#5045=ADVANCED_FACE ( 'NONE', ( #8451 ), #14927, .F. ) ;
#5056=ORIENTED_EDGE ( 'NONE', *, *, #14047, .T. ) ;
#5057=LINE ( 'NONE', #18604, #9901 ) ;
#5063=ORIENTED_EDGE ( 'NONE', *, *, #9219, .F. ) ;
#5064=DIRECTION ( 'NONE',  ( 0.000000000000000000, 0.000000000000000000, 1.000000000000000000 ) ) ;
#5070=EDGE_CURVE ( 'NONE', #7012, #15594, #20731, .T. ) ;
#5073=CARTESIAN_POINT ( 'NONE',  ( 30.00000000000000000, -105.0000000000000426, 77.45966692414833688 ) ) ;
#5077=VECTOR ( 'NONE', #2566, 1000.000000000000000 ) ;
#5081=DIRECTION ( 'NONE',  ( 1.000000000000000000, -0.000000000000000000, -0.000000000000000000 ) ) ;
#5084=AXIS2_PLACEMENT_3D ( 'NONE', #900, #7451, #10654 ) ;
#5087=EDGE_CURVE ( 'NONE', #4931, #20532, #17361, .T. ) ;
#5089=EDGE_CURVE ( 'NONE', #18338, #14577, #11232, .T. ) ;
#5090=CARTESIAN_POINT ( 'NONE',  ( 40.00000000000000711, -40.00000000000001421, -120.0000000000000142 ) ) ;
#5092=DIRECTION ( 'NONE',  ( 1.000000000000000000, -0.000000000000000000, -0.000000000000000000 ) ) ;
#5093=CARTESIAN_POINT ( 'NONE',  ( 43.13922815819793044, -11.21276953243446606, 82.40275014679680510 ) ) ;
#5095=ORIENTED_EDGE ( 'NONE', *, *, #17544, .F. ) ;
#5100=VERTEX_POINT ( 'NONE', #14083 ) ;
#5119=FACE_OUTER_BOUND ( 'NONE', #18132, .T. ) ;
#5125=CARTESIAN_POINT ( 'NONE',  ( -44.00000000000000000, -85.00000000000000000, -11.50000000000000711 ) ) ;
#5131=CIRCLE ( 'NONE', #8517, 39.99999999999999289 ) ;
#5134=AXIS2_PLACEMENT_3D ( 'NONE', #9527, #15997, #7947 ) ;
#5137=ORIENTED_EDGE ( 'NONE', *, *, #7204, .T. ) ;
#5139=EDGE_LOOP ( 'NONE', ( #15103, #16995, #18594, #10963 ) ) ;
#5144=VECTOR ( 'NONE', #16731, 1000.000000000000000 ) ;
#5148=ORIENTED_EDGE ( 'NONE', *, *, #17056, .F. ) ;
#5155=EDGE_CURVE ( 'NONE', #10337, #17904, #15765, .T. ) ;
#5157=VERTEX_POINT ( 'NONE', #20427 ) ;
#5159=DIRECTION ( 'NONE',  ( -1.000000000000000000, 0.000000000000000000, 0.000000000000000000 ) ) ;
#5162=CIRCLE ( 'NONE', #13306, 14.49999999999999467 ) ;
#5168=ORIENTED_EDGE ( 'NONE', *, *, #13304, .F. ) ;
#5169=EDGE_CURVE ( 'NONE', #18530, #20075, #873, .T. ) ;
#5170=ORIENTED_EDGE ( 'NONE', *, *, #16958, .F. ) ;
#5172=EDGE_CURVE ( 'NONE', #12906, #7841, #4325, .T. ) ;
#5177=AXIS2_PLACEMENT_3D ( 'NONE', #18174, #16367, #6714 ) ;
#5178=VECTOR ( 'NONE', #14671, 1000.000000000000000 ) ;
#5182=AXIS2_PLACEMENT_3D ( 'NONE', #10306, #18461, #5626 ) ;
#5191=LINE ( 'NONE', #8377, #13021 ) ;
#5194=VECTOR ( 'NONE', #12089, 1000.000000000000000 ) ;
#5199=EDGE_CURVE ( 'NONE', #4685, #14887, #19477, .T. ) ;
#5200=ORIENTED_EDGE ( 'NONE', *, *, #7570, .T. ) ;
#5206=( NAMED_UNIT ( * ) PLANE_ANGLE_UNIT ( ) SI_UNIT ( $, .RADIAN. ) );
#5216=CARTESIAN_POINT ( 'NONE',  ( 50.00000000000000000, 36.35083268962920044, -90.00000000000000000 ) ) ;
#5220=DIRECTION ( 'NONE',  ( 0.000000000000000000, -1.541976423090495387E-16, 1.000000000000000000 ) ) ;
#5221=EDGE_CURVE ( 'NONE', #13702, #19113, #3047, .T. ) ;
#5225=CIRCLE ( 'NONE', #7239, 8.500000000000000000 ) ;
#5229=CARTESIAN_POINT ( 'NONE',  ( 50.00000000000000000, 36.35083268962917202, 90.00000000000000000 ) ) ;
#5238=VERTEX_POINT ( 'NONE', #20843 ) ;
#5240=CARTESIAN_POINT ( 'NONE',  ( -24.99999999999999289, -160.0000000000000000, -53.99496054166690584 ) ) ;
#5242=EDGE_LOOP ( 'NONE', ( #13007, #14834, #10313, #11825 ) ) ;
#5243=DIRECTION ( 'NONE',  ( -1.000000000000000000, 0.000000000000000000, 0.000000000000000000 ) ) ;
#5247=DIRECTION ( 'NONE',  ( 0.000000000000000000, 0.000000000000000000, -1.000000000000000000 ) ) ;
#5251=DIRECTION ( 'NONE',  ( 1.000000000000000000, 0.000000000000000000, 0.000000000000000000 ) ) ;
#5254=ADVANCED_FACE ( 'NONE', ( #8123 ), #17980, .T. ) ;
#5256=DIRECTION ( 'NONE',  ( 0.000000000000000000, 0.000000000000000000, 1.000000000000000000 ) ) ;
#5265=AXIS2_PLACEMENT_3D ( 'NONE', #2894, #3002, #15823 ) ;
#5269=CARTESIAN_POINT ( 'NONE',  ( 36.56410540690647792, -119.8383876564256809, 84.69420751047145757 ) ) ;
#5271=ORIENTED_EDGE ( 'NONE', *, *, #11130, .T. ) ;
#5277=VERTEX_POINT ( 'NONE', #19358 ) ;
#5285=AXIS2_PLACEMENT_3D ( 'NONE', #20919, #4712, #1234 ) ;
#5294=ORIENTED_EDGE ( 'NONE', *, *, #13484, .F. ) ;
#5300=LINE ( 'NONE', #3803, #5194 ) ;
#5302=DIRECTION ( 'NONE',  ( 0.000000000000000000, 0.000000000000000000, -1.000000000000000000 ) ) ;
#5304=EDGE_LOOP ( 'NONE', ( #11435, #16240, #7271, #18294, #4348, #11997 ) ) ;
#5305=ORIENTED_EDGE ( 'NONE', *, *, #548, .F. ) ;
#5316=CARTESIAN_POINT ( 'NONE',  ( -23.00000000000000000, 2.816687638038912352E-15, -120.0000000000000142 ) ) ;
#5317=ADVANCED_FACE ( 'NONE', ( #6422 ), #4843, .F. ) ;
#5324=CARTESIAN_POINT ( 'NONE',  ( -11.54691128655044352, -18.15138880902594565, 72.10074112616622699 ) ) ;
#5343=CARTESIAN_POINT ( 'NONE',  ( -30.00000000000000000, -85.00000000000000000, -1.040949779275250179E-14 ) ) ;
#5350=VERTEX_POINT ( 'NONE', #13923 ) ;
#5358=EDGE_CURVE ( 'NONE', #5467, #19615, #12333, .T. ) ;
#5365=FACE_BOUND ( 'NONE', #5953, .T. ) ;
#5368=LINE ( 'NONE', #2401, #11227 ) ;
#5371=CARTESIAN_POINT ( 'NONE',  ( 32.39354794939547588, -114.5261895919207120, 81.05644908113433189 ) ) ;
#5373=ORIENTED_EDGE ( 'NONE', *, *, #4699, .F. ) ;
#5375=ORIENTED_EDGE ( 'NONE', *, *, #7907, .F. ) ;
#5380=CARTESIAN_POINT ( 'NONE',  ( 10.00000000000000178, -164.9999999999999716, 66.80000000000001137 ) ) ;
#5382=CARTESIAN_POINT ( 'NONE',  ( -24.99999999999999289, 31.35083268962915426, -50.63110039191615641 ) ) ;
#5387=EDGE_CURVE ( 'NONE', #15031, #9320, #14077, .T. ) ;
#5392=ORIENTED_EDGE ( 'NONE', *, *, #6286, .T. ) ;
#5397=DIRECTION ( 'NONE',  ( -1.000000000000000000, 0.000000000000000000, 0.000000000000000000 ) ) ;
#5398=CIRCLE ( 'NONE', #17266, 20.00000000000000000 ) ;
#5399=ORIENTED_EDGE ( 'NONE', *, *, #7137, .T. ) ;
#5400=CARTESIAN_POINT ( 'NONE',  ( 50.00000000000000000, -164.9999999999999716, -90.00000000000001421 ) ) ;
#5401=CARTESIAN_POINT ( 'NONE',  ( -21.50000000000000000, 0.000000000000000000, -68.00000000000000000 ) ) ;
#5402=VERTEX_POINT ( 'NONE', #18088 ) ;
#5404=CARTESIAN_POINT ( 'NONE',  ( 8.500000000000000000, 1.040949779275250140E-15, -81.99999999999998579 ) ) ;
#5406=LINE ( 'NONE', #18348, #3508 ) ;
#5408=VECTOR ( 'NONE', #652, 1000.000000000000000 ) ;
#5409=CARTESIAN_POINT ( 'NONE',  ( 32.40156131938952200, -114.5405781163270689, -81.06459374562506071 ) ) ;
#5410=CARTESIAN_POINT ( 'NONE',  ( -40.00000000000000000, 29.99999999999999289, -120.0000000000000142 ) ) ;
#5412=DIRECTION ( 'NONE',  ( 0.000000000000000000, 0.000000000000000000, -1.000000000000000000 ) ) ;
#5413=VERTEX_POINT ( 'NONE', #18477 ) ;
#5421=DIRECTION ( 'NONE',  ( -1.000000000000000000, 0.000000000000000000, 0.000000000000000000 ) ) ;
#5424=CARTESIAN_POINT ( 'NONE',  ( 45.76122707727121508, -127.3290820621008947, 85.00000000000000000 ) ) ;
#5429=CARTESIAN_POINT ( 'NONE',  ( 50.00000000000000000, 36.35083268962915781, 50.00000000000000000 ) ) ;
#5438=CARTESIAN_POINT ( 'NONE',  ( 10.15192380093073332, -18.95599582743659184, -71.71153801002554928 ) ) ;
#5439=VERTEX_POINT ( 'NONE', #7340 ) ;
#5443=ORIENTED_EDGE ( 'NONE', *, *, #15716, .F. ) ;
#5445=ORIENTED_EDGE ( 'NONE', *, *, #2623, .T. ) ;
#5447=ADVANCED_FACE ( 'NONE', ( #5745 ), #18687, .F. ) ;
#5453=AXIS2_PLACEMENT_3D ( 'NONE', #4680, #3298, #11241 ) ;
#5461=EDGE_CURVE ( 'NONE', #10995, #7518, #11257, .T. ) ;
#5462=CARTESIAN_POINT ( 'NONE',  ( -9.651484534775427448, -19.22442619234774241, 77.16801304840511477 ) ) ;
#5467=VERTEX_POINT ( 'NONE', #3207 ) ;
#5469=CARTESIAN_POINT ( 'NONE',  ( 30.87594499568497497, -110.8713507097124022, 79.29891132742112347 ) ) ;
#5479=ORIENTED_EDGE ( 'NONE', *, *, #5963, .T. ) ;
#5492=ORIENTED_EDGE ( 'NONE', *, *, #12703, .F. ) ;
#5498=DIRECTION ( 'NONE',  ( 0.000000000000000000, 0.000000000000000000, -1.000000000000000000 ) ) ;
#5499=VERTEX_POINT ( 'NONE', #9676 ) ;
#5502=ORIENTED_EDGE ( 'NONE', *, *, #18042, .F. ) ;
#5512=CARTESIAN_POINT ( 'NONE',  ( 35.38680890825803971, -118.6613745440660921, -83.76770575229788562 ) ) ;
#5513=DIRECTION ( 'NONE',  ( -0.000000000000000000, 0.000000000000000000, -1.000000000000000000 ) ) ;
#5514=VECTOR ( 'NONE', #1660, 1000.000000000000000 ) ;
#5517=AXIS2_PLACEMENT_3D ( 'NONE', #5090, #16027, #15916 ) ;
#5522=CARTESIAN_POINT ( 'NONE',  ( -12.15935632454279336, -17.74618724269112846, 72.30303056190481925 ) ) ;
#5524=LINE ( 'NONE', #7221, #11941 ) ;
#5533=LINE ( 'NONE', #578, #7024 ) ;
#5542=CARTESIAN_POINT ( 'NONE',  ( -44.00000000000000000, -85.00000000000000000, 14.49999999999998579 ) ) ;
#5546=CARTESIAN_POINT ( 'NONE',  ( 15.62350230547614416, -14.77425901644549278, -73.92464627053527693 ) ) ;
#5547=ORIENTED_EDGE ( 'NONE', *, *, #16642, .F. ) ;
#5549=FACE_OUTER_BOUND ( 'NONE', #7876, .T. ) ;
#5550=LINE ( 'NONE', #2282, #1259 ) ;
#5552=ORIENTED_EDGE ( 'NONE', *, *, #10912, .F. ) ;
#5556=VERTEX_POINT ( 'NONE', #10947 ) ;
#5558=EDGE_LOOP ( 'NONE', ( #3066, #2977 ) ) ;
#5563=EDGE_CURVE ( 'NONE', #14001, #8060, #19119, .T. ) ;
#5566=DIRECTION ( 'NONE',  ( 0.000000000000000000, 0.000000000000000000, -1.000000000000000000 ) ) ;
#5567=CARTESIAN_POINT ( 'NONE',  ( -9.017423154539844887, -19.53047022166475699, 77.00824986274105299 ) ) ;
#5569=CARTESIAN_POINT ( 'NONE',  ( 23.13963350654227824, -26.35784117651622793, -120.0000000000000142 ) ) ;
#5570=ADVANCED_FACE ( 'NONE', ( #1532 ), #3100, .T. ) ;
#5577=CARTESIAN_POINT ( 'NONE',  ( -1.485268882270375679, -22.96492952317579395, -75.38826545565814286 ) ) ;
#5586=DIRECTION ( 'NONE',  ( -1.000000000000000000, 0.000000000000000000, 0.000000000000000000 ) ) ;
#5589=EDGE_CURVE ( 'NONE', #20286, #14728, #19823, .T. ) ;
#5591=VECTOR ( 'NONE', #17427, 1000.000000000000000 ) ;
#5596=AXIS2_PLACEMENT_3D ( 'NONE', #1710, #11243, #9548 ) ;
#5604=DIRECTION ( 'NONE',  ( 0.000000000000000000, 0.000000000000000000, 1.000000000000000000 ) ) ;
#5610=CARTESIAN_POINT ( 'NONE',  ( 45.22159793441011999, -8.673994507468391291, -78.07221698934968401 ) ) ;
#5617=AXIS2_PLACEMENT_3D ( 'NONE', #16739, #9088, #933 ) ;
#5626=DIRECTION ( 'NONE',  ( 1.000000000000000000, 0.000000000000000000, 0.000000000000000000 ) ) ;
#5633=EDGE_LOOP ( 'NONE', ( #1364, #18096, #13595, #18836 ) ) ;
#5635=CARTESIAN_POINT ( 'NONE',  ( -20.48001470518130418, -6.654962914332833712, 79.70582905289666087 ) ) ;
#5641=AXIS2_PLACEMENT_3D ( 'NONE', #14213, #10916, #15894 ) ;
#5656=CARTESIAN_POINT ( 'NONE',  ( -12.15935632454278625, -17.74618724269114622, -72.30303056190483346 ) ) ;
#5658=EDGE_CURVE ( 'NONE', #231, #5157, #12961, .T. ) ;
#5663=ORIENTED_EDGE ( 'NONE', *, *, #11143, .T. ) ;
#5665=DIRECTION ( 'NONE',  ( 0.000000000000000000, 0.000000000000000000, -1.000000000000000000 ) ) ;
#5666=EDGE_LOOP ( 'NONE', ( #2723, #15129, #3200, #14766, #3981, #15027, #19429 ) ) ;
#5669=FACE_OUTER_BOUND ( 'NONE', #8609, .T. ) ;
#5670=DIRECTION ( 'NONE',  ( -1.000000000000000000, -0.000000000000000000, -0.000000000000000000 ) ) ;
#5678=CARTESIAN_POINT ( 'NONE',  ( -18.23093333169988739, -11.40057928256656439, 82.28885341040493984 ) ) ;
#5684=VERTEX_POINT ( 'NONE', #5007 ) ;
#5686=DIRECTION ( 'NONE',  ( 0.000000000000000000, 0.000000000000000000, 1.000000000000000000 ) ) ;
#5687=VERTEX_POINT ( 'NONE', #6786 ) ;
#5693=CARTESIAN_POINT ( 'NONE',  ( 45.22159793441013420, -8.673994507468389514, -84.62946326583126222 ) ) ;
#5703=DIRECTION ( 'NONE',  ( -1.000000000000000000, -0.000000000000000000, -0.000000000000000000 ) ) ;
#5711=CARTESIAN_POINT ( 'NONE',  ( -24.99999999999999289, -85.00000000000000000, 74.99999999999998579 ) ) ;
#5714=CARTESIAN_POINT ( 'NONE',  ( 36.29350642860042342, -22.37888450698892484, -70.21894222985346801 ) ) ;
#5731=EDGE_CURVE ( 'NONE', #7518, #13187, #12050, .T. ) ;
#5732=ORIENTED_EDGE ( 'NONE', *, *, #18089, .T. ) ;
#5736=CARTESIAN_POINT ( 'NONE',  ( 14.60954982181483963, -15.77788197283120120, 73.35099031848520212 ) ) ;
#5745=FACE_OUTER_BOUND ( 'NONE', #8298, .T. ) ;
#5755=VERTEX_POINT ( 'NONE', #8480 ) ;
#5756=CARTESIAN_POINT ( 'NONE',  ( 17.61872475889259704, -12.39310755016574817, -75.38263485905285677 ) ) ;
#5759=FACE_OUTER_BOUND ( 'NONE', #7158, .T. ) ;
#5762=CARTESIAN_POINT ( 'NONE',  ( -24.99999999999999645, -85.00000000000000000, -1.040949779275250179E-14 ) ) ;
#5764=LINE ( 'NONE', #13945, #10221 ) ;
#5772=EDGE_CURVE ( 'NONE', #18485, #13263, #8385, .T. ) ;
#5779=CARTESIAN_POINT ( 'NONE',  ( -20.81434048145373339, -5.479059011584746841, 87.82828572917365761 ) ) ;
#5789=CARTESIAN_POINT ( 'NONE',  ( 30.00000000000000000, -122.0000000000000000, -2.099999999999997424 ) ) ;
#5793=VERTEX_POINT ( 'NONE', #5404 ) ;
#5794=ORIENTED_EDGE ( 'NONE', *, *, #9338, .F. ) ;
#5796=AXIS2_PLACEMENT_3D ( 'NONE', #14734, #16011, #211 ) ;
#5797=VECTOR ( 'NONE', #8019, 1000.000000000000000 ) ;
#5801=DIRECTION ( 'NONE',  ( 1.000000000000000000, 0.000000000000000000, 0.000000000000000000 ) ) ;
#5809=EDGE_CURVE ( 'NONE', #2556, #14202, #13482, .T. ) ;
#5811=CARTESIAN_POINT ( 'NONE',  ( 11.50000000000000000, 0.000000000000000000, 81.99999999999998579 ) ) ;
#5815=CARTESIAN_POINT ( 'NONE',  ( 40.00000000000000711, 39.99999999999998579, -130.0000000000000000 ) ) ;
#5817=CARTESIAN_POINT ( 'NONE',  ( -27.96694501150314593, -24.74873734152930993, -120.0000000000000142 ) ) ;
#5820=EDGE_CURVE ( 'NONE', #18485, #7631, #6622, .T. ) ;
#5822=ORIENTED_EDGE ( 'NONE', *, *, #12206, .T. ) ;
#5830=AXIS2_PLACEMENT_3D ( 'NONE', #4345, #738, #7623 ) ;
#5832=CARTESIAN_POINT ( 'NONE',  ( 0.000000000000000000, 0.000000000000000000, -130.0000000000000000 ) ) ;
#5841=VERTEX_POINT ( 'NONE', #3809 ) ;
#5842=DIRECTION ( 'NONE',  ( -1.000000000000000000, -0.000000000000000000, -0.000000000000000000 ) ) ;
#5843=ORIENTED_EDGE ( 'NONE', *, *, #4093, .T. ) ;
#5853=CARTESIAN_POINT ( 'NONE',  ( 43.74543371413037107, -125.0989072405818661, 82.69023214352036177 ) ) ;
#5855=LINE ( 'NONE', #20265, #1301 ) ;
#5861=CARTESIAN_POINT ( 'NONE',  ( 46.54332301554113371, -6.983203288388278196, 86.24273042526077404 ) ) ;
#5868=VECTOR ( 'NONE', #20149, 1000.000000000000000 ) ;
#5869=VERTEX_POINT ( 'NONE', #6998 ) ;
#5877=EDGE_LOOP ( 'NONE', ( #9809, #584, #17386, #4043 ) ) ;
#5879=CARTESIAN_POINT ( 'NONE',  ( 50.00000000000000000, -159.9999999999999716, 85.00000000000000000 ) ) ;
#5882=ORIENTED_EDGE ( 'NONE', *, *, #9510, .F. ) ;
#5884=VECTOR ( 'NONE', #3109, 1000.000000000000000 ) ;
#5886=ORIENTED_EDGE ( 'NONE', *, *, #8367, .T. ) ;
#5889=CIRCLE ( 'NONE', #17742, 10.00000000000000178 ) ;
#5890=AXIS2_PLACEMENT_3D ( 'NONE', #7652, #20365, #14133 ) ;
#5901=VECTOR ( 'NONE', #14744, 1000.000000000000000 ) ;
#5908=EDGE_LOOP ( 'NONE', ( #3174, #18509 ) ) ;
#5909=CARTESIAN_POINT ( 'NONE',  ( 12.30490414407268851, -19.44545088549631018, -77.05113792083442092 ) ) ;
#5910=CARTESIAN_POINT ( 'NONE',  ( -24.99999999999999289, -97.49621075554985339, 111.6458212409894486 ) ) ;
#5916=FACE_OUTER_BOUND ( 'NONE', #2888, .T. ) ;
#5928=VERTEX_POINT ( 'NONE', #8904 ) ;
#5929=ADVANCED_FACE ( 'NONE', ( #10500 ), #13576, .T. ) ;
#5942=VECTOR ( 'NONE', #3953, 1000.000000000000000 ) ;
#5943=FACE_OUTER_BOUND ( 'NONE', #1843, .T. ) ;
#5953=EDGE_LOOP ( 'NONE', ( #15822, #3823 ) ) ;
#5961=ORIENTED_EDGE ( 'NONE', *, *, #15174, .F. ) ;
#5963=EDGE_CURVE ( 'NONE', #1568, #17751, #15378, .T. ) ;
#5965=LINE ( 'NONE', #15606, #3595 ) ;
#5973=AXIS2_PLACEMENT_3D ( 'NONE', #11717, #19654, #14895 ) ;
#5977=EDGE_LOOP ( 'NONE', ( #10687, #4226 ) ) ;
#5978=DIRECTION ( 'NONE',  ( -1.000000000000000000, -0.000000000000000000, -0.000000000000000000 ) ) ;
#6000=ORIENTED_EDGE ( 'NONE', *, *, #13718, .T. ) ;
#6001=FACE_OUTER_BOUND ( 'NONE', #16252, .T. ) ;
#6011=EDGE_CURVE ( 'NONE', #7012, #5684, #10025, .T. ) ;
#6014=AXIS2_PLACEMENT_3D ( 'NONE', #12484, #13755, #4526 ) ;
#6015=ORIENTED_EDGE ( 'NONE', *, *, #2600, .T. ) ;
#6016=DIRECTION ( 'NONE',  ( -1.000000000000000000, -0.000000000000000000, -0.000000000000000000 ) ) ;
#6019=AXIS2_PLACEMENT_3D ( 'NONE', #17655, #14781, #9699 ) ;
#6020=EDGE_CURVE ( 'NONE', #3970, #19211, #11133, .T. ) ;
#6030=EDGE_LOOP ( 'NONE', ( #718, #7106, #9632, #6000, #12254, #17389 ) ) ;
#6031=CARTESIAN_POINT ( 'NONE',  ( -30.00000000000000000, -125.0000000000000000, 90.00000000000002842 ) ) ;
#6033=DIRECTION ( 'NONE',  ( 0.000000000000000000, 0.000000000000000000, 1.000000000000000000 ) ) ;
#6041=CARTESIAN_POINT ( 'NONE',  ( 33.28744621271695792, -29.52989836050402772, -73.00509023842178635 ) ) ;
#6044=ORIENTED_EDGE ( 'NONE', *, *, #6381, .T. ) ;
#6045=CARTESIAN_POINT ( 'NONE',  ( 30.84620721615401351, -110.7731078431028777, -73.91085715544664936 ) ) ;
#6046=CARTESIAN_POINT ( 'NONE',  ( 50.00000000000000000, 31.35083268962917558, 84.99999999999998579 ) ) ;
#6047=ADVANCED_FACE ( 'NONE', ( #7521 ), #15794, .F. ) ;
#6048=EDGE_CURVE ( 'NONE', #2608, #14851, #17395, .T. ) ;
#6054=ORIENTED_EDGE ( 'NONE', *, *, #12607, .F. ) ;
#6059=ORIENTED_EDGE ( 'NONE', *, *, #17772, .T. ) ;
#6084=DIRECTION ( 'NONE',  ( 0.000000000000000000, 0.000000000000000000, -1.000000000000000000 ) ) ;
#6087=EDGE_CURVE ( 'NONE', #4783, #6177, #7842, .T. ) ;
#6089=EDGE_CURVE ( 'NONE', #16461, #15306, #9018, .T. ) ;
#6097=CARTESIAN_POINT ( 'NONE',  ( 18.81636376335696426, -10.41831967068597997, 83.08843782764408559 ) ) ;
#6102=CIRCLE ( 'NONE', #6775, 5.000000000000000888 ) ;
#6105=EDGE_CURVE ( 'NONE', #14994, #9313, #414, .T. ) ;
#6107=CARTESIAN_POINT ( 'NONE',  ( 30.00000000000000000, -99.99999999999998579, -52.00000000000000000 ) ) ;
#6130=ORIENTED_EDGE ( 'NONE', *, *, #672, .F. ) ;
#6134=CYLINDRICAL_SURFACE ( 'NONE', #12786, 2.099999999999997868 ) ;
#6136=DIRECTION ( 'NONE',  ( 0.000000000000000000, 0.000000000000000000, -1.000000000000000000 ) ) ;
#6139=CARTESIAN_POINT ( 'NONE',  ( -30.00000000000000000, -49.99999999999997868, 71.93747284969079203 ) ) ;
#6149=AXIS2_PLACEMENT_3D ( 'NONE', #1372, #7724, #7817 ) ;
#6153=DIRECTION ( 'NONE',  ( 0.000000000000000000, 0.000000000000000000, -1.000000000000000000 ) ) ;
#6154=CARTESIAN_POINT ( 'NONE',  ( -24.99999999999999289, 31.35083268962909742, -2.067608244099269852E-13 ) ) ;
#6155=ORIENTED_EDGE ( 'NONE', *, *, #5589, .F. ) ;
#6157=ORIENTED_EDGE ( 'NONE', *, *, #15380, .T. ) ;
#6162=ORIENTED_EDGE ( 'NONE', *, *, #9944, .T. ) ;
#6163=DIRECTION ( 'NONE',  ( 0.000000000000000000, 0.000000000000000000, -1.000000000000000000 ) ) ;
#6167=VERTEX_POINT ( 'NONE', #19692 ) ;
#6171=AXIS2_PLACEMENT_3D ( 'NONE', #10566, #11939, #13443 ) ;
#6177=VERTEX_POINT ( 'NONE', #13238 ) ;
#6182=CARTESIAN_POINT ( 'NONE',  ( -44.00000000000000000, -85.00000000000000000, 11.49999999999998579 ) ) ;
#6186=ORIENTED_EDGE ( 'NONE', *, *, #18434, .T. ) ;
#6199=AXIS2_PLACEMENT_3D ( 'NONE', #262, #16264, #10007 ) ;
#6200=EDGE_CURVE ( 'NONE', #20704, #4938, #18167, .T. ) ;
#6205=DIRECTION ( 'NONE',  ( 0.000000000000000000, 0.000000000000000000, 1.000000000000000000 ) ) ;
#6209=CARTESIAN_POINT ( 'NONE',  ( 15.31456654470125400, -15.09377138507804972, 79.61049916633108126 ) ) ;
#6210=AXIS2_PLACEMENT_3D ( 'NONE', #13381, #15170, #977 ) ;
#6216=DIRECTION ( 'NONE',  ( -1.000000000000000000, 0.000000000000000000, 0.000000000000000000 ) ) ;
#6219=CIRCLE ( 'NONE', #14690, 54.99999999999999289 ) ;
#6234=ORIENTED_EDGE ( 'NONE', *, *, #585, .F. ) ;
#6235=CARTESIAN_POINT ( 'NONE',  ( -30.00000000000000000, 36.35083268962920044, -90.00000000000000000 ) ) ;
#6242=CARTESIAN_POINT ( 'NONE',  ( 21.18805271706017024, -3.649167310370820871, 90.00000000000000000 ) ) ;
#6244=EDGE_CURVE ( 'NONE', #17375, #18530, #8150, .T. ) ;
#6252=CARTESIAN_POINT ( 'NONE',  ( 45.22159793441011999, -8.673994507468391291, -78.07221698934968401 ) ) ;
#6254=EDGE_CURVE ( 'NONE', #15415, #20612, #7743, .T. ) ;
#6256=CARTESIAN_POINT ( 'NONE',  ( 50.00000000000000000, 36.35083268962917202, 90.00000000000000000 ) ) ;
#6258=CARTESIAN_POINT ( 'NONE',  ( -30.00000000000000000, 36.35083268962920044, -90.00000000000000000 ) ) ;
#6265=VERTEX_POINT ( 'NONE', #3783 ) ;
#6266=DIRECTION ( 'NONE',  ( 0.000000000000000000, 0.000000000000000000, 1.000000000000000000 ) ) ;
#6272=EDGE_CURVE ( 'NONE', #3394, #7841, #6967, .T. ) ;
#6276=DIRECTION ( 'NONE',  ( 0.000000000000000000, -0.000000000000000000, -1.000000000000000000 ) ) ;
#6286=EDGE_CURVE ( 'NONE', #18936, #20567, #8559, .T. ) ;
#6294=DIRECTION ( 'NONE',  ( 0.000000000000000000, 0.000000000000000000, -1.000000000000000000 ) ) ;
#6299=ORIENTED_EDGE ( 'NONE', *, *, #14660, .F. ) ;
#6311=ADVANCED_FACE ( 'NONE', ( #13456 ), #20106, .F. ) ;
#6321=ORIENTED_EDGE ( 'NONE', *, *, #2110, .T. ) ;
#6326=CARTESIAN_POINT ( 'NONE',  ( -15.68987849063190687, -16.83236858365102506, -78.51413802123066432 ) ) ;
#6337=VECTOR ( 'NONE', #11309, 1000.000000000000000 ) ;
#6338=CIRCLE ( 'NONE', #18189, 2.099999999999997868 ) ;
#6339=CARTESIAN_POINT ( 'NONE',  ( -30.00000000000000000, -124.9999999999999858, -90.00000000000001421 ) ) ;
#6342=CARTESIAN_POINT ( 'NONE',  ( 39.99999999999999289, -122.3205080756887639, -86.97287527660684248 ) ) ;
#6343=CIRCLE ( 'NONE', #6014, 20.00000000000000000 ) ;
#6352=DIRECTION ( 'NONE',  ( 0.000000000000000000, 0.000000000000000000, -1.000000000000000000 ) ) ;
#6368=DIRECTION ( 'NONE',  ( 0.000000000000000000, 0.000000000000000000, -1.000000000000000000 ) ) ;
#6378=ORIENTED_EDGE ( 'NONE', *, *, #9106, .F. ) ;
#6381=EDGE_CURVE ( 'NONE', #4041, #3394, #1605, .T. ) ;
#6389=EDGE_CURVE ( 'NONE', #5687, #5684, #1370, .T. ) ;
#6396=DIRECTION ( 'NONE',  ( 1.000000000000000000, -0.000000000000000000, -0.000000000000000000 ) ) ;
#6397=EDGE_CURVE ( 'NONE', #14667, #17074, #11062, .T. ) ;
#6401=DIRECTION ( 'NONE',  ( 1.000000000000000000, 0.000000000000000000, 0.000000000000000000 ) ) ;
#6402=ORIENTED_EDGE ( 'NONE', *, *, #5658, .F. ) ;
#6412=CARTESIAN_POINT ( 'NONE',  ( 6.991428239010133439, -20.34384952674291469, 76.59572168033703576 ) ) ;
#6413=CYLINDRICAL_SURFACE ( 'NONE', #18316, 20.00000000000000000 ) ;
#6422=FACE_OUTER_BOUND ( 'NONE', #15793, .T. ) ;
#6426=DIRECTION ( 'NONE',  ( 0.000000000000000000, -1.000000000000000000, 0.000000000000000000 ) ) ;
#6432=CARTESIAN_POINT ( 'NONE',  ( -24.99999999999999289, -85.00000000000000000, -1.040949779275250179E-14 ) ) ;
#6443=ORIENTED_EDGE ( 'NONE', *, *, #7260, .F. ) ;
#6444=DIRECTION ( 'NONE',  ( 1.000000000000000000, 0.000000000000000000, 0.000000000000000000 ) ) ;
#6448=ORIENTED_EDGE ( 'NONE', *, *, #17544, .T. ) ;
#6450=CARTESIAN_POINT ( 'NONE',  ( 49.19234958605026264, -1.326995226329880762, -84.99999999999998579 ) ) ;
#6451=VECTOR ( 'NONE', #6153, 1000.000000000000000 ) ;
#6460=DIRECTION ( 'NONE',  ( -1.000000000000000000, -0.000000000000000000, -0.000000000000000000 ) ) ;
#6464=ORIENTED_EDGE ( 'NONE', *, *, #8501, .T. ) ;
#6466=CARTESIAN_POINT ( 'NONE',  ( -30.00000000000000000, -164.9999999999999716, -50.00000000000000711 ) ) ;
#6467=AXIS2_PLACEMENT_3D ( 'NONE', #5400, #855, #20017 ) ;
#6468=EDGE_LOOP ( 'NONE', ( #11111, #16484, #4913, #3071 ) ) ;
#6481=AXIS2_PLACEMENT_3D ( 'NONE', #4974, #19590, #5064 ) ;
#6482=ORIENTED_EDGE ( 'NONE', *, *, #5221, .T. ) ;
#6488=DIRECTION ( 'NONE',  ( 1.000000000000000000, -0.000000000000000000, -0.000000000000000000 ) ) ;
#6503=CARTESIAN_POINT ( 'NONE',  ( 38.52090548607635867, -121.4001261175067299, 79.56756026429930273 ) ) ;
#6504=EDGE_CURVE ( 'NONE', #20567, #19615, #14143, .T. ) ;
#6511=ADVANCED_FACE ( 'NONE', ( #13976 ), #18748, .T. ) ;
#6522=ORIENTED_EDGE ( 'NONE', *, *, #3897, .T. ) ;
#6524=DIRECTION ( 'NONE',  ( -0.000000000000000000, -0.000000000000000000, 1.000000000000000000 ) ) ;
#6525=CIRCLE ( 'NONE', #18378, 11.50000000000000000 ) ;
#6536=ORIENTED_EDGE ( 'NONE', *, *, #17056, .T. ) ;
#6538=VECTOR ( 'NONE', #14784, 1000.000000000000000 ) ;
#6551=ORIENTED_EDGE ( 'NONE', *, *, #5221, .F. ) ;
#6552=CARTESIAN_POINT ( 'NONE',  ( 24.99999999999999645, -85.00000000000000000, -1.040949779275250179E-14 ) ) ;
#6556=CARTESIAN_POINT ( 'NONE',  ( -24.99999999999999289, 230.0000000000000000, 85.00000000000000000 ) ) ;
#6570=AXIS2_PLACEMENT_3D ( 'NONE', #11359, #17833, #3306 ) ;
#6571=ORIENTED_EDGE ( 'NONE', *, *, #3510, .F. ) ;
#6575=VERTEX_POINT ( 'NONE', #1773 ) ;
#6577=VERTEX_POINT ( 'NONE', #19467 ) ;
#6579=CARTESIAN_POINT ( 'NONE',  ( 30.88247860994248128, -39.30399960665665304, -66.45597419381263649 ) ) ;
#6584=AXIS2_PLACEMENT_3D ( 'NONE', #4724, #17768, #16174 ) ;
#6586=ORIENTED_EDGE ( 'NONE', *, *, #6989, .F. ) ;
#6598=EDGE_CURVE ( 'NONE', #10440, #15031, #9725, .T. ) ;
#6600=VERTEX_POINT ( 'NONE', #12817 ) ;
#6604=EDGE_LOOP ( 'NONE', ( #15534, #12368, #19118, #4759, #2555, #6988, #8450 ) ) ;
#6610=ORIENTED_EDGE ( 'NONE', *, *, #6254, .F. ) ;
#6614=CARTESIAN_POINT ( 'NONE',  ( -20.80121494421295125, -5.547499958777468265, -80.68520720011532887 ) ) ;
#6621=EDGE_LOOP ( 'NONE', ( #14914, #14976, #20483, #6798, #14427, #18165, #15575, #8711, #2382 ) ) ;
#6622=CIRCLE ( 'NONE', #9016, 75.00000000000001421 ) ;
#6626=FACE_OUTER_BOUND ( 'NONE', #20409, .T. ) ;
#6628=CIRCLE ( 'NONE', #16787, 23.00000000000000000 ) ;
#6635=DIRECTION ( 'NONE',  ( 0.000000000000000000, 0.000000000000000000, -1.000000000000000000 ) ) ;
#6647=EDGE_CURVE ( 'NONE', #12774, #5100, #3613, .T. ) ;
#6649=FACE_OUTER_BOUND ( 'NONE', #20796, .T. ) ;
#6652=EDGE_CURVE ( 'NONE', #7841, #5402, #4976, .T. ) ;
#6653=AXIS2_PLACEMENT_3D ( 'NONE', #15820, #1319, #9253 ) ;
#6654=CARTESIAN_POINT ( 'NONE',  ( -30.00000000000000000, -49.99999999999999289, -71.93747284969079203 ) ) ;
#6655=FACE_OUTER_BOUND ( 'NONE', #14318, .T. ) ;
#6662=ORIENTED_EDGE ( 'NONE', *, *, #5070, .T. ) ;
#6664=CARTESIAN_POINT ( 'NONE',  ( 49.01761906262722590, -1.923047794321506743, -84.32426567686945873 ) ) ;
#6666=AXIS2_PLACEMENT_3D ( 'NONE', #10167, #5703, #7080 ) ;
#6674=CARTESIAN_POINT ( 'NONE',  ( -22.96694501150314238, -24.74873734152930993, -120.0000000000000142 ) ) ;
#6683=ORIENTED_EDGE ( 'NONE', *, *, #4027, .F. ) ;
#6685=CARTESIAN_POINT ( 'NONE',  ( 38.31677532819030318, -18.47596261708826049, 77.53674502934073587 ) ) ;
#6686=ORIENTED_EDGE ( 'NONE', *, *, #10468, .T. ) ;
#6691=ADVANCED_FACE ( 'NONE', ( #17682, #9723 ), #3153, .F. ) ;
#6694=CARTESIAN_POINT ( 'NONE',  ( 30.00000000000000000, -39.99999999999999289, -49.89999999999999858 ) ) ;
#6699=FACE_OUTER_BOUND ( 'NONE', #5877, .T. ) ;
#6702=DIRECTION ( 'NONE',  ( 0.000000000000000000, 0.000000000000000000, -1.000000000000000000 ) ) ;
#6709=ORIENTED_EDGE ( 'NONE', *, *, #5563, .T. ) ;
#6714=DIRECTION ( 'NONE',  ( 0.000000000000000000, 0.000000000000000000, -1.000000000000000000 ) ) ;
#6720=ORIENTED_EDGE ( 'NONE', *, *, #1444, .T. ) ;
#6727=EDGE_CURVE ( 'NONE', #14851, #5277, #16485, .T. ) ;
#6732=CARTESIAN_POINT ( 'NONE',  ( -24.99999999999999645, -97.49621075554985339, -111.6458212409894486 ) ) ;
#6737=EDGE_CURVE ( 'NONE', #7841, #12500, #11826, .T. ) ;
#6738=EDGE_LOOP ( 'NONE', ( #12513, #9495, #2577, #11492, #15522, #19616 ) ) ;
#6741=PLANE ( 'NONE',  #16179 ) ;
#6744=CARTESIAN_POINT ( 'NONE',  ( 50.00000000000000000, 31.35083268962912584, 6.892027480330899929E-14 ) ) ;
#6745=EDGE_CURVE ( 'NONE', #15579, #15761, #18398, .T. ) ;
#6746=EDGE_CURVE ( 'NONE', #1213, #16235, #14483, .T. ) ;
#6750=DIRECTION ( 'NONE',  ( 1.000000000000000000, 0.000000000000000000, 0.000000000000000000 ) ) ;
#6754=ORIENTED_EDGE ( 'NONE', *, *, #12098, .T. ) ;
#6756=CYLINDRICAL_SURFACE ( 'NONE', #15679, 8.500000000000000000 ) ;
#6760=CARTESIAN_POINT ( 'NONE',  ( 47.02940313615643220, -6.215498114345216152, 80.10634491168215732 ) ) ;
#6764=DIRECTION ( 'NONE',  ( 1.000000000000000000, 0.000000000000000000, 0.000000000000000000 ) ) ;
#6766=DIRECTION ( 'NONE',  ( -1.000000000000000000, 0.000000000000000000, 0.000000000000000000 ) ) ;
#6773=ORIENTED_EDGE ( 'NONE', *, *, #14493, .T. ) ;
#6775=AXIS2_PLACEMENT_3D ( 'NONE', #7878, #136, #1428 ) ;
#6777=LINE ( 'NONE', #4997, #1185 ) ;
#6779=CARTESIAN_POINT ( 'NONE',  ( -30.00000000000000000, -85.00000000000000000, -1.040949779275250179E-14 ) ) ;
#6780=EDGE_LOOP ( 'NONE', ( #5170, #4635, #15686, #6443, #18775 ) ) ;
#6784=AXIS2_PLACEMENT_3D ( 'NONE', #14852, #5092, #13057 ) ;
#6786=CARTESIAN_POINT ( 'NONE',  ( 30.00000000000000000, -105.0000000000000000, -77.45966692414833688 ) ) ;
#6790=CARTESIAN_POINT ( 'NONE',  ( 34.82290702564237961, -118.0320511495591802, -83.30093209484321903 ) ) ;
#6796=EDGE_CURVE ( 'NONE', #15340, #2130, #15322, .T. ) ;
#6798=ORIENTED_EDGE ( 'NONE', *, *, #1972, .T. ) ;
#6801=VERTEX_POINT ( 'NONE', #3974 ) ;
#6802=DIRECTION ( 'NONE',  ( -1.000000000000000000, 0.000000000000000000, 0.000000000000000000 ) ) ;
#6804=DIRECTION ( 'NONE',  ( 1.000000000000000000, 0.000000000000000000, 0.000000000000000000 ) ) ;
#6809=AXIS2_PLACEMENT_3D ( 'NONE', #18531, #6856, #622 ) ;
#6813=AXIS2_PLACEMENT_3D ( 'NONE', #20668, #1402, #16125 ) ;
#6817=ORIENTED_EDGE ( 'NONE', *, *, #10110, .F. ) ;
#6831=CYLINDRICAL_SURFACE ( 'NONE', #8212, 11.50000000000000000 ) ;
#6841=EDGE_LOOP ( 'NONE', ( #2363, #6709, #17969, #2131 ) ) ;
#6842=DIRECTION ( 'NONE',  ( 0.000000000000000000, 0.000000000000000000, -1.000000000000000000 ) ) ;
#6843=VERTEX_POINT ( 'NONE', #10344 ) ;
#6845=DIRECTION ( 'NONE',  ( 0.000000000000000000, 0.000000000000000000, 1.000000000000000000 ) ) ;
#6846=AXIS2_PLACEMENT_3D ( 'NONE', #810, #15216, #13845 ) ;
#6847=ORIENTED_EDGE ( 'NONE', *, *, #11447, .T. ) ;
#6856=DIRECTION ( 'NONE',  ( -0.000000000000000000, -0.000000000000000000, -1.000000000000000000 ) ) ;
#6858=EDGE_CURVE ( 'NONE', #20725, #18615, #2296, .T. ) ;
#6861=CARTESIAN_POINT ( 'NONE',  ( 48.03213166600498596, -4.380080863984868067, -81.79793649453739590 ) ) ;
#6867=CIRCLE ( 'NONE', #3819, 8.500000000000000000 ) ;
#6876=CIRCLE ( 'NONE', #1158, 80.00000000000000000 ) ;
#6885=CIRCLE ( 'NONE', #5890, 21.50000000000000000 ) ;
#6887=DIRECTION ( 'NONE',  ( 1.000000000000000000, 0.000000000000000000, 0.000000000000000000 ) ) ;
#6895=EDGE_CURVE ( 'NONE', #17074, #9451, #8963, .T. ) ;
#6906=ADVANCED_FACE ( 'NONE', ( #9076 ), #14266, .F. ) ;
#6907=ORIENTED_EDGE ( 'NONE', *, *, #4006, .T. ) ;
#6909=ORIENTED_EDGE ( 'NONE', *, *, #6895, .T. ) ;
#6911=CARTESIAN_POINT ( 'NONE',  ( -30.00000000000000000, 230.0000000000000000, 0.000000000000000000 ) ) ;
#6912=VECTOR ( 'NONE', #16243, 1000.000000000000000 ) ;
#6913=EDGE_LOOP ( 'NONE', ( #20867, #15781, #18576, #5961 ) ) ;
#6920=CIRCLE ( 'NONE', #16728, 8.500000000000000000 ) ;
#6921=CARTESIAN_POINT ( 'NONE',  ( 0.000000000000000000, 0.000000000000000000, -68.00000000000000000 ) ) ;
#6925=DIRECTION ( 'NONE',  ( 0.000000000000000000, 0.000000000000000000, -1.000000000000000000 ) ) ;
#6928=DIRECTION ( 'NONE',  ( 1.000000000000000000, 0.000000000000000000, 0.000000000000000000 ) ) ;
#6930=ORIENTED_EDGE ( 'NONE', *, *, #13950, .F. ) ;
#6931=LINE ( 'NONE', #16573, #3040 ) ;
#6932=AXIS2_PLACEMENT_3D ( 'NONE', #14888, #363, #13302 ) ;
#6937=ORIENTED_EDGE ( 'NONE', *, *, #14701, .T. ) ;
#6941=LINE ( 'NONE', #3659, #16671 ) ;
#6958=CARTESIAN_POINT ( 'NONE',  ( 0.000000000000000000, 0.000000000000000000, -130.0000000000000000 ) ) ;
#6960=ORIENTED_EDGE ( 'NONE', *, *, #8419, .F. ) ;
#6963=DIRECTION ( 'NONE',  ( -0.000000000000000000, 0.000000000000000000, -1.000000000000000000 ) ) ;
#6967=LINE ( 'NONE', #15456, #16802 ) ;
#6978=AXIS2_PLACEMENT_3D ( 'NONE', #574, #884, #17098 ) ;
#6986=DIRECTION ( 'NONE',  ( 0.000000000000000000, 0.000000000000000000, 1.000000000000000000 ) ) ;
#6988=ORIENTED_EDGE ( 'NONE', *, *, #9224, .F. ) ;
#6989=EDGE_CURVE ( 'NONE', #12782, #5350, #11027, .T. ) ;
#6994=CARTESIAN_POINT ( 'NONE',  ( 43.37263506394752000, -10.84340913432649600, -76.37419715032000056 ) ) ;
#6998=CARTESIAN_POINT ( 'NONE',  ( -21.50000000000000000, 0.000000000000000000, -84.99999999999998579 ) ) ;
#7004=VECTOR ( 'NONE', #4653, 1000.000000000000000 ) ;
#7006=AXIS2_PLACEMENT_3D ( 'NONE', #12289, #1060, #14796 ) ;
#7007=EDGE_CURVE ( 'NONE', #8524, #7867, #3428, .T. ) ;
#7008=DIRECTION ( 'NONE',  ( -1.000000000000000000, 0.000000000000000000, 0.000000000000000000 ) ) ;
#7012=VERTEX_POINT ( 'NONE', #14486 ) ;
#7017=CARTESIAN_POINT ( 'NONE',  ( 2.985015299703225100, -21.29524168283704810, 70.66569055735612892 ) ) ;
#7021=ORIENTED_EDGE ( 'NONE', *, *, #4880, .F. ) ;
#7024=VECTOR ( 'NONE', #472, 1000.000000000000000 ) ;
#7027=EDGE_CURVE ( 'NONE', #10438, #5556, #19544, .T. ) ;
#7028=CARTESIAN_POINT ( 'NONE',  ( -44.00000000000000000, -85.00000000000000000, -1.040949779275250179E-14 ) ) ;
#7035=EDGE_CURVE ( 'NONE', #15733, #10469, #19219, .T. ) ;
#7038=CARTESIAN_POINT ( 'NONE',  ( 18.66082225198900701, -10.69875493221381113, -76.55584491636109590 ) ) ;
#7042=FACE_OUTER_BOUND ( 'NONE', #13254, .T. ) ;
#7049=DIRECTION ( 'NONE',  ( -1.000000000000000000, 0.000000000000000000, 0.000000000000000000 ) ) ;
#7059=ORIENTED_EDGE ( 'NONE', *, *, #20198, .F. ) ;
#7060=EDGE_CURVE ( 'NONE', #6600, #20805, #1951, .T. ) ;
#7061=CARTESIAN_POINT ( 'NONE',  ( 33.28482093211906800, -115.9902465777789047, 81.92806195354719989 ) ) ;
#7068=ORIENTED_EDGE ( 'NONE', *, *, #26, .F. ) ;
#7069=ORIENTED_EDGE ( 'NONE', *, *, #15174, .T. ) ;
#7078=APPLICATION_CONTEXT ( 'automotive_design' ) ;
#7080=DIRECTION ( 'NONE',  ( 0.000000000000000000, 0.000000000000000000, 1.000000000000000000 ) ) ;
#7085=CARTESIAN_POINT ( 'NONE',  ( 8.500000000000000000, 0.000000000000000000, 81.99999999999998579 ) ) ;
#7091=CARTESIAN_POINT ( 'NONE',  ( 39.22505056128680678, -16.94578504268678287, -72.69725825150482024 ) ) ;
#7098=FACE_OUTER_BOUND ( 'NONE', #7535, .T. ) ;
#7102=CARTESIAN_POINT ( 'NONE',  ( 32.00705917571151815, -113.7759157576893898, -80.64955526189534396 ) ) ;
#7106=ORIENTED_EDGE ( 'NONE', *, *, #7204, .F. ) ;
#7110=CARTESIAN_POINT ( 'NONE',  ( 1.457308041610579474, -21.46427008073575493, 70.59507481315790756 ) ) ;
#7113=CARTESIAN_POINT ( 'NONE',  ( 30.00000000000000711, 29.99999999999998579, -120.0000000000000142 ) ) ;
#7116=DIRECTION ( 'NONE',  ( -1.000000000000000000, 0.000000000000000000, 0.000000000000000000 ) ) ;
#7121=AXIS2_PLACEMENT_3D ( 'NONE', #5343, #3738, #11711 ) ;
#7131=CARTESIAN_POINT ( 'NONE',  ( 13.80207632871712775, -16.50074880709950165, -72.95245019206021198 ) ) ;
#7135=CYLINDRICAL_SURFACE ( 'NONE', #20188, 50.00000000000001421 ) ;
#7137=EDGE_CURVE ( 'NONE', #9883, #11773, #19555, .T. ) ;
#7140=DIRECTION ( 'NONE',  ( 0.000000000000000000, 0.000000000000000000, 1.000000000000000000 ) ) ;
#7146=ORIENTED_EDGE ( 'NONE', *, *, #10925, .F. ) ;
#7150=CARTESIAN_POINT ( 'NONE',  ( 30.00000000000000000, -85.00000000000000000, -1.040949779275250179E-14 ) ) ;
#7153=VECTOR ( 'NONE', #19967, 1000.000000000000000 ) ;
#7158=EDGE_LOOP ( 'NONE', ( #12754, #18336, #5305, #375 ) ) ;
#7164=ORIENTED_EDGE ( 'NONE', *, *, #15265, .F. ) ;
#7165=DIRECTION ( 'NONE',  ( 0.000000000000000000, 0.000000000000000000, -1.000000000000000000 ) ) ;
#7169=CARTESIAN_POINT ( 'NONE',  ( 9.319588655241851427, -21.03063704226208941, -76.26165510927667412 ) ) ;
#7177=DIRECTION ( 'NONE',  ( -1.000000000000000000, -0.000000000000000000, -0.000000000000000000 ) ) ;
#7181=EDGE_CURVE ( 'NONE', #10552, #8802, #1639, .T. ) ;
#7190=LINE ( 'NONE', #9214, #1107 ) ;
#7198=ORIENTED_EDGE ( 'NONE', *, *, #19805, .T. ) ;
#7201=AXIS2_PLACEMENT_3D ( 'NONE', #11705, #3640, #50 ) ;
#7203=CARTESIAN_POINT ( 'NONE',  ( 50.00000000000000000, 230.0000000000000000, 85.00000000000000000 ) ) ;
#7204=EDGE_CURVE ( 'NONE', #5238, #19472, #18197, .T. ) ;
#7214=AXIS2_PLACEMENT_3D ( 'NONE', #9770, #120, #1718 ) ;
#7216=CARTESIAN_POINT ( 'NONE',  ( 50.00000000000000000, -177.4842959289096029, -65.62505536500324865 ) ) ;
#7217=ORIENTED_EDGE ( 'NONE', *, *, #3673, .F. ) ;
#7219=CARTESIAN_POINT ( 'NONE',  ( -19.00859264729084330, -10.06624177801188758, 77.01193977728054563 ) ) ;
#7221=CARTESIAN_POINT ( 'NONE',  ( 50.00000000000000000, -42.57363661491096707, -66.38288848018790134 ) ) ;
#7226=ORIENTED_EDGE ( 'NONE', *, *, #17562, .F. ) ;
#7237=DIRECTION ( 'NONE',  ( 0.000000000000000000, 0.000000000000000000, 1.000000000000000000 ) ) ;
#7239=AXIS2_PLACEMENT_3D ( 'NONE', #9465, #17216, #4485 ) ;
#7240=CARTESIAN_POINT ( 'NONE',  ( -0.8281006575391230973, -21.49753944123813909, -70.58133206268969673 ) ) ;
#7243=ADVANCED_FACE ( 'NONE', ( #5119 ), #3637, .F. ) ;
#7245=CARTESIAN_POINT ( 'NONE',  ( 50.00000000000000000, -170.8299878242309546, -15.48896927112552824 ) ) ;
#7247=ORIENTED_EDGE ( 'NONE', *, *, #8561, .F. ) ;
#7248=PLANE ( 'NONE',  #16337 ) ;
#7251=LINE ( 'NONE', #10338, #7505 ) ;
#7252=EDGE_CURVE ( 'NONE', #12463, #13263, #5533, .T. ) ;
#7254=CYLINDRICAL_SURFACE ( 'NONE', #17022, 75.00000000000000000 ) ;
#7256=DIRECTION ( 'NONE',  ( 1.000000000000000000, 0.000000000000000000, 0.000000000000000000 ) ) ;
#7257=CARTESIAN_POINT ( 'NONE',  ( -44.00000000000000000, -85.00000000000000000, -1.040949779275250179E-14 ) ) ;
#7260=EDGE_CURVE ( 'NONE', #2149, #17375, #18371, .T. ) ;
#7263=DIRECTION ( 'NONE',  ( -1.000000000000000000, 0.000000000000000000, 0.000000000000000000 ) ) ;
#7271=ORIENTED_EDGE ( 'NONE', *, *, #12468, .F. ) ;
#7273=CARTESIAN_POINT ( 'NONE',  ( 31.99811442804358208, -113.7578330439423269, 80.63997760446149243 ) ) ;
#7276=CARTESIAN_POINT ( 'NONE',  ( 14.12295668597094078, -18.21227605178592057, -77.70918423292295074 ) ) ;
#7282=VERTEX_POINT ( 'NONE', #20051 ) ;
#7283=CARTESIAN_POINT ( 'NONE',  ( 46.54332301554112661, -6.983203288388267538, -86.24273042526071720 ) ) ;
#7286=LINE ( 'NONE', #18859, #16315 ) ;
#7295=CARTESIAN_POINT ( 'NONE',  ( 30.00000000000000000, -85.00000000000000000, -1.040949779275250179E-14 ) ) ;
#7312=DIRECTION ( 'NONE',  ( 1.000000000000000000, 0.000000000000000000, 0.000000000000000000 ) ) ;
#7314=DIRECTION ( 'NONE',  ( 0.000000000000000000, 0.000000000000000000, 1.000000000000000000 ) ) ;
#7316=CARTESIAN_POINT ( 'NONE',  ( 0.000000000000000000, 0.000000000000000000, 68.00000000000000000 ) ) ;
#7330=CARTESIAN_POINT ( 'NONE',  ( 3.744012722225321443, -21.17498532244396614, 70.71631193418075156 ) ) ;
#7332=EDGE_CURVE ( 'NONE', #3623, #12159, #5965, .T. ) ;
#7340=CARTESIAN_POINT ( 'NONE',  ( -24.99999999999999289, -84.99999999999998579, -75.00000000000001421 ) ) ;
#7344=CARTESIAN_POINT ( 'NONE',  ( 30.43430782549248903, -42.57363661491096707, -66.38288848018790134 ) ) ;
#7349=ORIENTED_EDGE ( 'NONE', *, *, #6858, .T. ) ;
#7351=CARTESIAN_POINT ( 'NONE',  ( -24.99999999999999289, -40.41646384503850697, -66.42520834682601105 ) ) ;
#7353=CARTESIAN_POINT ( 'NONE',  ( 15.37884418493265848, -15.02891098528240654, -73.77646566961475116 ) ) ;
#7354=ORIENTED_EDGE ( 'NONE', *, *, #12600, .F. ) ;
#7355=VECTOR ( 'NONE', #9393, 1000.000000000000000 ) ;
#7361=CARTESIAN_POINT ( 'NONE',  ( 50.00000000000000000, -127.3290820621008947, 85.00000000000000000 ) ) ;
#7380=CARTESIAN_POINT ( 'NONE',  ( 0.000000000000000000, 0.000000000000000000, -90.00000000000000000 ) ) ;
#7381=CARTESIAN_POINT ( 'NONE',  ( 30.00000000000000000, -110.0000000000000142, 44.99999999999999289 ) ) ;
#7383=CARTESIAN_POINT ( 'NONE',  ( 30.00000000000000000, -39.99999999999999289, 49.89999999999999858 ) ) ;
#7384=ORIENTED_EDGE ( 'NONE', *, *, #4497, .T. ) ;
#7392=EDGE_CURVE ( 'NONE', #1631, #13026, #20180, .T. ) ;
#7394=LINE ( 'NONE', #15663, #19372 ) ;
#7405=EDGE_LOOP ( 'NONE', ( #14396, #5399, #331, #2666 ) ) ;
#7408=CARTESIAN_POINT ( 'NONE',  ( 30.00000000000000000, -47.51018795805313033, -71.56352010304497924 ) ) ;
#7411=EDGE_CURVE ( 'NONE', #15579, #4783, #17313, .T. ) ;
#7416=ORIENTED_EDGE ( 'NONE', *, *, #12825, .F. ) ;
#7418=DIRECTION ( 'NONE',  ( -0.000000000000000000, -0.000000000000000000, 1.000000000000000000 ) ) ;
#7421=EDGE_CURVE ( 'NONE', #4938, #20704, #13137, .T. ) ;
#7425=CARTESIAN_POINT ( 'NONE',  ( 43.62500077266424370, -124.9999999999999858, -90.00000000000001421 ) ) ;
#7427=DIRECTION ( 'NONE',  ( 1.000000000000000000, 0.000000000000000000, 0.000000000000000000 ) ) ;
#7428=AXIS2_PLACEMENT_3D ( 'NONE', #15536, #15221, #9085 ) ;
#7429=ORIENTED_EDGE ( 'NONE', *, *, #14933, .T. ) ;
#7433=CARTESIAN_POINT ( 'NONE',  ( 0.000000000000000000, 0.000000000000000000, 81.99999999999998579 ) ) ;
#7435=EDGE_CURVE ( 'NONE', #2489, #18656, #8998, .T. ) ;
#7450=ADVANCED_FACE ( 'NONE', ( #1802 ), #16217, .F. ) ;
#7451=DIRECTION ( 'NONE',  ( -0.000000000000000000, -1.000000000000000000, -0.000000000000000000 ) ) ;
#7453=CARTESIAN_POINT ( 'NONE',  ( 7.417002224176414416, -20.23665979631132572, -71.11836349014900804 ) ) ;
#7454=DIRECTION ( 'NONE',  ( -1.000000000000000000, 0.000000000000000000, 0.000000000000000000 ) ) ;
#7465=VECTOR ( 'NONE', #3926, 1000.000000000000000 ) ;
#7468=PRODUCT ( 'Sealed Cast Iron Gearbox Casing', 'Sealed Cast Iron Gearbox Casing', '', ( #12041 ) ) ;
#7481=LINE ( 'NONE', #10168, #17143 ) ;
#7482=ORIENTED_EDGE ( 'NONE', *, *, #3851, .F. ) ;
#7486=CARTESIAN_POINT ( 'NONE',  ( 20.50516414656735265, -10.42283242499551932, -83.08857956002572109 ) ) ;
#7501=EDGE_LOOP ( 'NONE', ( #5168, #13481, #12119, #15282, #3134 ) ) ;
#7504=CARTESIAN_POINT ( 'NONE',  ( -39.99999999999999289, -40.00000000000000000, -130.0000000000000000 ) ) ;
#7505=VECTOR ( 'NONE', #20285, 1000.000000000000000 ) ;
#7518=VERTEX_POINT ( 'NONE', #19597 ) ;
#7521=FACE_OUTER_BOUND ( 'NONE', #6604, .T. ) ;
#7525=AXIS2_PLACEMENT_3D ( 'NONE', #19371, #14717, #17800 ) ;
#7527=AXIS2_PLACEMENT_3D ( 'NONE', #16279, #19771, #172 ) ;
#7530=CYLINDRICAL_SURFACE ( 'NONE', #15967, 63.70999227554992217 ) ;
#7531=AXIS2_PLACEMENT_3D ( 'NONE', #4079, #5566, #7263 ) ;
#7533=DIRECTION ( 'NONE',  ( 0.000000000000000000, -0.000000000000000000, 1.000000000000000000 ) ) ;
#7535=EDGE_LOOP ( 'NONE', ( #15768, #15963, #20845, #515 ) ) ;
#7536=CYLINDRICAL_SURFACE ( 'NONE', #19347, 80.00000000000000000 ) ;
#7537=EDGE_CURVE ( 'NONE', #2306, #2910, #16311, .T. ) ;
#7542=EDGE_LOOP ( 'NONE', ( #16685, #3780 ) ) ;
#7553=DIRECTION ( 'NONE',  ( -0.000000000000000000, 0.000000000000000000, -1.000000000000000000 ) ) ;
#7559=VECTOR ( 'NONE', #8809, 1000.000000000000000 ) ;
#7566=LINE ( 'NONE', #6182, #2160 ) ;
#7570=EDGE_CURVE ( 'NONE', #8121, #11513, #12118, .T. ) ;
#7579=ORIENTED_EDGE ( 'NONE', *, *, #15982, .F. ) ;
#7581=VECTOR ( 'NONE', #5397, 1000.000000000000000 ) ;
#7584=CARTESIAN_POINT ( 'NONE',  ( 32.99516560860324432, -115.5366112665960259, 75.94268391876913427 ) ) ;
#7585=DIRECTION ( 'NONE',  ( 0.000000000000000000, 1.000000000000000000, 0.000000000000000000 ) ) ;
#7598=EDGE_LOOP ( 'NONE', ( #13936, #16162, #9913, #16785 ) ) ;
#7599=DIRECTION ( 'NONE',  ( 0.000000000000000000, 0.000000000000000000, -1.000000000000000000 ) ) ;
#7602=CARTESIAN_POINT ( 'NONE',  ( 17.19937875120477955, -15.27427100821770800, -79.49209680402589129 ) ) ;
#7604=DIRECTION ( 'NONE',  ( -1.000000000000000000, 0.000000000000000000, 0.000000000000000000 ) ) ;
#7619=B_SPLINE_CURVE_WITH_KNOTS ( 'NONE', 3,
 ( #17065, #7408, #7625, #12616 ),
 .UNSPECIFIED., .F., .F.,
 ( 4, 4 ),
 ( 2.797157557069881010E-17, 0.007433635558789152172 ),
 .UNSPECIFIED. ) ;
#7620=CARTESIAN_POINT ( 'NONE',  ( 50.00000000000000000, -170.8299878242309546, 15.48896927112552824 ) ) ;
#7623=DIRECTION ( 'NONE',  ( 0.000000000000000000, 0.000000000000000000, -1.000000000000000000 ) ) ;
#7625=CARTESIAN_POINT ( 'NONE',  ( 30.14545621897691774, -45.03477164951879530, -71.38288848018790134 ) ) ;
#7629=CARTESIAN_POINT ( 'NONE',  ( 37.09297593336772536, -20.77527980508516592, -76.37819121560252711 ) ) ;
#7631=VERTEX_POINT ( 'NONE', #11645 ) ;
#7633=CARTESIAN_POINT ( 'NONE',  ( 39.62131026106984422, -122.1018714529781022, -80.10792010848122402 ) ) ;
#7642=LINE ( 'NONE', #4137, #4762 ) ;
#7650=CARTESIAN_POINT ( 'NONE',  ( 50.00000000000000000, -160.0000000000000000, 79.59486983196745769 ) ) ;
#7652=CARTESIAN_POINT ( 'NONE',  ( 0.000000000000000000, 0.000000000000000000, -84.99999999999998579 ) ) ;
#7660=CARTESIAN_POINT ( 'NONE',  ( 30.00000000000000000, -99.99999999999998579, 54.09999999999999432 ) ) ;
#7664=FACE_OUTER_BOUND ( 'NONE', #18368, .T. ) ;
#7671=AXIS2_PLACEMENT_3D ( 'NONE', #8244, #14720, #17996 ) ;
#7680=EDGE_LOOP ( 'NONE', ( #16156, #17318, #6683, #13375, #11865, #20156, #332, #20677 ) ) ;
#7683=CARTESIAN_POINT ( 'NONE',  ( -39.99999999999999289, -40.00000000000000000, -120.0000000000000142 ) ) ;
#7685=VERTEX_POINT ( 'NONE', #18752 ) ;
#7688=ORIENTED_EDGE ( 'NONE', *, *, #5199, .F. ) ;
#7689=CARTESIAN_POINT ( 'NONE',  ( -39.99999999999999289, -30.00000000000000000, -120.0000000000000142 ) ) ;
#7694=CIRCLE ( 'NONE', #2624, 21.50000000000000000 ) ;
#7698=DIRECTION ( 'NONE',  ( -1.000000000000000000, 0.000000000000000000, 0.000000000000000000 ) ) ;
#7702=LINE ( 'NONE', #9493, #9977 ) ;
#7703=AXIS2_PLACEMENT_3D ( 'NONE', #17340, #20614, #1133 ) ;
#7706=CARTESIAN_POINT ( 'NONE',  ( 13.11093970363753769, -17.09443977129685521, 78.35293316767238991 ) ) ;
#7707=CIRCLE ( 'NONE', #8703, 80.00000000000000000 ) ;
#7717=DIRECTION ( 'NONE',  ( 1.000000000000000000, 0.000000000000000000, 0.000000000000000000 ) ) ;
#7722=DIRECTION ( 'NONE',  ( -0.000000000000000000, -1.000000000000000000, -0.000000000000000000 ) ) ;
#7723=FACE_BOUND ( 'NONE', #11819, .T. ) ;
#7724=DIRECTION ( 'NONE',  ( 0.000000000000000000, 0.000000000000000000, -1.000000000000000000 ) ) ;
#7732=EDGE_CURVE ( 'NONE', #16753, #2149, #4294, .T. ) ;
#7737=ORIENTED_EDGE ( 'NONE', *, *, #9219, .T. ) ;
#7740=CARTESIAN_POINT ( 'NONE',  ( -24.99999999999999289, -85.00000000000000000, -1.040949779275250179E-14 ) ) ;
#7742=EDGE_LOOP ( 'NONE', ( #569, #20791, #1445, #6571 ) ) ;
#7743=B_SPLINE_CURVE_WITH_KNOTS ( 'NONE', 3,
 ( #20216, #15140, #12164, #7283, #8989, #5693 ),
 .UNSPECIFIED., .F., .F.,
 ( 4, 2, 4 ),
 ( 0.000000000000000000, 0.003996741055817027918, 0.007993482111634055837 ),
 .UNSPECIFIED. ) ;
#7747=LINE ( 'NONE', #6258, #3758 ) ;
#7753=CARTESIAN_POINT ( 'NONE',  ( 0.000000000000000000, 0.000000000000000000, 84.99999999999998579 ) ) ;
#7773=CARTESIAN_POINT ( 'NONE',  ( -31.35784117651625635, 26.35784117651607872, -130.0000000000000000 ) ) ;
#7782=DIRECTION ( 'NONE',  ( 1.000000000000000000, 0.000000000000000000, 0.000000000000000000 ) ) ;
#7783=ORIENTED_EDGE ( 'NONE', *, *, #18170, .T. ) ;
#7784=EDGE_CURVE ( 'NONE', #7685, #20241, #398, .T. ) ;
#7787=FACE_OUTER_BOUND ( 'NONE', #19741, .T. ) ;
#7788=ADVANCED_FACE ( 'NONE', ( #12069, #13869 ), #20316, .F. ) ;
#7798=ORIENTED_EDGE ( 'NONE', *, *, #6089, .F. ) ;
#7799=CARTESIAN_POINT ( 'NONE',  ( 5.636490946615987596, -20.76011204682435718, 76.39151275260617524 ) ) ;
#7810=CARTESIAN_POINT ( 'NONE',  ( 50.00000000000000000, 36.35083268962917202, 90.00000000000000000 ) ) ;
#7815=CARTESIAN_POINT ( 'NONE',  ( 0.000000000000000000, 0.000000000000000000, -120.0000000000000142 ) ) ;
#7817=DIRECTION ( 'NONE',  ( -1.000000000000000000, 0.000000000000000000, 0.000000000000000000 ) ) ;
#7818=CARTESIAN_POINT ( 'NONE',  ( 41.41808208302015970, -123.1392381480534226, 87.79662768828310959 ) ) ;
#7824=DIRECTION ( 'NONE',  ( 0.000000000000000000, 1.000000000000000000, 1.040834085586084454E-15 ) ) ;
#7825=ADVANCED_FACE ( 'NONE', ( #9420 ), #1273, .T. ) ;
#7831=CARTESIAN_POINT ( 'NONE',  ( 8.500000000000000000, 0.000000000000000000, 81.99999999999998579 ) ) ;
#7838=FACE_OUTER_BOUND ( 'NONE', #20308, .T. ) ;
#7839=ORIENTED_EDGE ( 'NONE', *, *, #6020, .T. ) ;
#7841=VERTEX_POINT ( 'NONE', #14295 ) ;
#7842=LINE ( 'NONE', #14324, #14464 ) ;
#7846=CARTESIAN_POINT ( 'NONE',  ( 39.99999999999999289, -122.3205080756887639, -86.97287527660684248 ) ) ;
#7855=CARTESIAN_POINT ( 'NONE',  ( 24.99999999999999645, -99.99999999999998579, 54.09999999999999432 ) ) ;
#7857=FACE_OUTER_BOUND ( 'NONE', #16580, .T. ) ;
#7860=DIRECTION ( 'NONE',  ( -1.000000000000000000, 0.000000000000000000, 0.000000000000000000 ) ) ;
#7865=CARTESIAN_POINT ( 'NONE',  ( 50.00000000000000000, 230.0000000000000000, 84.99999999999998579 ) ) ;
#7867=VERTEX_POINT ( 'NONE', #14088 ) ;
#7876=EDGE_LOOP ( 'NONE', ( #1819, #4800, #13756, #13839 ) ) ;
#7878=CARTESIAN_POINT ( 'NONE',  ( 23.13963350654227824, -26.35784117651622793, -130.0000000000000000 ) ) ;
#7879=ORIENTED_EDGE ( 'NONE', *, *, #18675, .F. ) ;
#7885=CARTESIAN_POINT ( 'NONE',  ( 24.74873734152916072, 24.74873734152916072, -120.0000000000000142 ) ) ;
#7890=ORIENTED_EDGE ( 'NONE', *, *, #1711, .F. ) ;
#7896=DIRECTION ( 'NONE',  ( 0.000000000000000000, 0.000000000000000000, -1.000000000000000000 ) ) ;
#7907=EDGE_CURVE ( 'NONE', #8783, #18257, #7251, .T. ) ;
#7909=VERTEX_POINT ( 'NONE', #12358 ) ;
#7911=VECTOR ( 'NONE', #19267, 1000.000000000000000 ) ;
#7912=CARTESIAN_POINT ( 'NONE',  ( 24.99999999999999645, -30.00000000000000711, -1.040949779275250179E-14 ) ) ;
#7916=ORIENTED_EDGE ( 'NONE', *, *, #13741, .F. ) ;
#7920=DIRECTION ( 'NONE',  ( 1.000000000000000000, -0.000000000000000000, -0.000000000000000000 ) ) ;
#7934=CIRCLE ( 'NONE', #8256, 14.49999999999999467 ) ;
#7935=ADVANCED_FACE ( 'NONE', ( #17123 ), #4187, .F. ) ;
#7942=ORIENTED_EDGE ( 'NONE', *, *, #12088, .T. ) ;
#7947=DIRECTION ( 'NONE',  ( 0.000000000000000000, 0.000000000000000000, -1.000000000000000000 ) ) ;
#7948=EDGE_LOOP ( 'NONE', ( #2686, #5056, #183, #12325, #12620, #19594, #16025, #3226 ) ) ;
#7950=FACE_BOUND ( 'NONE', #16680, .T. ) ;
#7954=EDGE_LOOP ( 'NONE', ( #5095, #303, #6015, #11317, #18027 ) ) ;
#7956=EDGE_CURVE ( 'NONE', #20282, #4158, #690, .T. ) ;
#7957=EDGE_CURVE ( 'NONE', #2701, #12906, #912, .T. ) ;
#7960=CYLINDRICAL_SURFACE ( 'NONE', #8233, 23.00000000000000000 ) ;
#7967=CYLINDRICAL_SURFACE ( 'NONE', #10706, 14.49999999999999467 ) ;
#7985=LINE ( 'NONE', #19223, #11976 ) ;
#7986=ORIENTED_EDGE ( 'NONE', *, *, #12317, .T. ) ;
#7990=ORIENTED_EDGE ( 'NONE', *, *, #5589, .T. ) ;
#7994=ORIENTED_EDGE ( 'NONE', *, *, #1991, .T. ) ;
#7995=EDGE_CURVE ( 'NONE', #9883, #4283, #5764, .T. ) ;
#7997=CARTESIAN_POINT ( 'NONE',  ( 10.00000000000000178, -164.9999999999999716, 73.20000000000000284 ) ) ;
#8000=CARTESIAN_POINT ( 'NONE',  ( 0.000000000000000000, 0.000000000000000000, -68.00000000000000000 ) ) ;
#8018=VECTOR ( 'NONE', #4096, 1000.000000000000000 ) ;
#8019=DIRECTION ( 'NONE',  ( 0.000000000000000000, -1.000000000000000000, 0.000000000000000000 ) ) ;
#8020=CARTESIAN_POINT ( 'NONE',  ( 0.000000000000000000, 0.000000000000000000, -68.00000000000000000 ) ) ;
#8023=ORIENTED_EDGE ( 'NONE', *, *, #6244, .T. ) ;
#8031=AXIS2_PLACEMENT_3D ( 'NONE', #539, #6986, #13474 ) ;
#8033=CARTESIAN_POINT ( 'NONE',  ( 0.000000000000000000, 0.000000000000000000, 81.99999999999998579 ) ) ;
#8043=LINE ( 'NONE', #18965, #7004 ) ;
#8045=DIRECTION ( 'NONE',  ( 1.000000000000000000, 0.000000000000000000, 0.000000000000000000 ) ) ;
#8046=CIRCLE ( 'NONE', #18194, 2.099999999999990763 ) ;
#8054=CARTESIAN_POINT ( 'NONE',  ( 0.000000000000000000, 0.000000000000000000, 90.00000000000000000 ) ) ;
#8057=FACE_OUTER_BOUND ( 'NONE', #7680, .T. ) ;
#8058=DIRECTION ( 'NONE',  ( 0.000000000000000000, 0.000000000000000000, 1.000000000000000000 ) ) ;
#8060=VERTEX_POINT ( 'NONE', #7689 ) ;
#8061=ORIENTED_EDGE ( 'NONE', *, *, #585, .T. ) ;
#8065=EDGE_CURVE ( 'NONE', #17850, #9196, #11178, .T. ) ;
#8070=LINE ( 'NONE', #3191, #1752 ) ;
#8071=EDGE_CURVE ( 'NONE', #5402, #16359, #4815, .T. ) ;
#8081=DIRECTION ( 'NONE',  ( 1.000000000000000000, 0.000000000000000000, 0.000000000000000000 ) ) ;
#8082=ORIENTED_EDGE ( 'NONE', *, *, #6989, .T. ) ;
#8083=DIRECTION ( 'NONE',  ( -1.000000000000000000, 0.000000000000000000, 0.000000000000000000 ) ) ;
#8084=CARTESIAN_POINT ( 'NONE',  ( 41.14327188351807507, -13.96402716752546169, 80.34089272068401044 ) ) ;
#8086=EDGE_LOOP ( 'NONE', ( #12766, #11412 ) ) ;
#8091=FACE_OUTER_BOUND ( 'NONE', #17998, .T. ) ;
#8094=DIRECTION ( 'NONE',  ( 0.000000000000000000, 0.000000000000000000, -1.000000000000000000 ) ) ;
#8096=DIRECTION ( 'NONE',  ( 0.000000000000000000, 0.7812527682501551052, 0.6242147964454778375 ) ) ;
#8102=ORIENTED_EDGE ( 'NONE', *, *, #6381, .F. ) ;
#8103=CARTESIAN_POINT ( 'NONE',  ( -30.00000000000000000, 36.35083268962917202, 90.00000000000000000 ) ) ;
#8105=DIRECTION ( 'NONE',  ( 0.000000000000000000, 1.000000000000000000, 0.000000000000000000 ) ) ;
#8106=ORIENTED_EDGE ( 'NONE', *, *, #13101, .T. ) ;
#8115=DIRECTION ( 'NONE',  ( 0.000000000000000000, 0.000000000000000000, 1.000000000000000000 ) ) ;
#8120=CARTESIAN_POINT ( 'NONE',  ( 30.00000000000000000, -105.0000000000000000, -90.00000000000001421 ) ) ;
#8121=VERTEX_POINT ( 'NONE', #19028 ) ;
#8123=FACE_OUTER_BOUND ( 'NONE', #6780, .T. ) ;
#8126=DIRECTION ( 'NONE',  ( 1.000000000000000000, 0.000000000000000000, 0.000000000000000000 ) ) ;
#8134=CARTESIAN_POINT ( 'NONE',  ( 50.00000000000000000, 31.35083268962909742, -2.067608244099269852E-13 ) ) ;
#8141=CARTESIAN_POINT ( 'NONE',  ( 38.67130833460402073, -17.89826649859318408, 72.22104433765980502 ) ) ;
#8146=DIRECTION ( 'NONE',  ( 0.000000000000000000, 0.000000000000000000, 1.000000000000000000 ) ) ;
#8150=LINE ( 'NONE', #6556, #577 ) ;
#8152=CIRCLE ( 'NONE', #8807, 11.49999999999999645 ) ;
#8162=DIRECTION ( 'NONE',  ( 0.000000000000000000, 0.000000000000000000, -1.000000000000000000 ) ) ;
#8164=ORIENTED_EDGE ( 'NONE', *, *, #20339, .T. ) ;
#8169=ADVANCED_FACE ( 'NONE', ( #7787 ), #14060, .T. ) ;
#8174=CARTESIAN_POINT ( 'NONE',  ( 30.62662295113251787, -40.93503228410152417, -66.38288848018791555 ) ) ;
#8179=CARTESIAN_POINT ( 'NONE',  ( 49.19234958605026264, -1.326995226329880762, -84.99999999999998579 ) ) ;
#8198=DIRECTION ( 'NONE',  ( 0.000000000000000000, 0.000000000000000000, 1.000000000000000000 ) ) ;
#8209=CYLINDRICAL_SURFACE ( 'NONE', #1861, 21.50000000000000000 ) ;
#8211=CARTESIAN_POINT ( 'NONE',  ( 45.22159793441011999, -8.673994507468391291, -78.07221698934968401 ) ) ;
#8212=AXIS2_PLACEMENT_3D ( 'NONE', #3447, #8525, #8327 ) ;
#8216=FACE_OUTER_BOUND ( 'NONE', #18658, .T. ) ;
#8217=CYLINDRICAL_SURFACE ( 'NONE', #3929, 10.00000000000000178 ) ;
#8220=LINE ( 'NONE', #8120, #1277 ) ;
#8222=VECTOR ( 'NONE', #17765, 1000.000000000000000 ) ;
#8223=DIRECTION ( 'NONE',  ( 0.000000000000000000, 1.000000000000000000, 1.040834085586084454E-15 ) ) ;
#8228=DIRECTION ( 'NONE',  ( 1.000000000000000000, 0.000000000000000000, 0.000000000000000000 ) ) ;
#8229=PLANE ( 'NONE',  #11269 ) ;
#8233=AXIS2_PLACEMENT_3D ( 'NONE', #11235, #3291, #13149 ) ;
#8235=DIRECTION ( 'NONE',  ( 1.000000000000000000, 0.000000000000000000, 0.000000000000000000 ) ) ;
#8242=EDGE_CURVE ( 'NONE', #15031, #4041, #14838, .T. ) ;
#8244=CARTESIAN_POINT ( 'NONE',  ( 0.000000000000000000, 0.000000000000000000, -68.00000000000000000 ) ) ;
#8245=CARTESIAN_POINT ( 'NONE',  ( 32.99404949636548423, -30.67485788781106848, 67.67723498345976907 ) ) ;
#8246=EDGE_LOOP ( 'NONE', ( #16793, #16831, #717, #20150 ) ) ;
#8248=DIRECTION ( 'NONE',  ( 0.000000000000000000, 1.000000000000000000, 0.000000000000000000 ) ) ;
#8249=VERTEX_POINT ( 'NONE', #5382 ) ;
#8251=CARTESIAN_POINT ( 'NONE',  ( 24.99999999999999645, -99.99999999999998579, -49.89999999999999858 ) ) ;
#8253=EDGE_LOOP ( 'NONE', ( #590, #15134, #11903, #11400 ) ) ;
#8256=AXIS2_PLACEMENT_3D ( 'NONE', #13184, #9888, #8401 ) ;
#8262=AXIS2_PLACEMENT_3D ( 'NONE', #2690, #128, #14652 ) ;
#8268=ORIENTED_EDGE ( 'NONE', *, *, #4439, .F. ) ;
#8271=CARTESIAN_POINT ( 'NONE',  ( 30.00000000000000000, -39.99999999999999289, 54.09999999999999432 ) ) ;
#8273=CARTESIAN_POINT ( 'NONE',  ( 45.22159793441011999, -8.673994507468384185, 84.62946326583127643 ) ) ;
#8274=VERTEX_POINT ( 'NONE', #13553 ) ;
#8280=EDGE_CURVE ( 'NONE', #6577, #3526, #10063, .T. ) ;
#8281=CARTESIAN_POINT ( 'NONE',  ( 50.00000000000000000, 31.35083268962909742, -2.067608244099269852E-13 ) ) ;
#8298=EDGE_LOOP ( 'NONE', ( #8552, #8949, #13841, #13503 ) ) ;
#8304=ADVANCED_FACE ( 'NONE', ( #9565 ), #524, .T. ) ;
#8306=CARTESIAN_POINT ( 'NONE',  ( 37.16069494243885885, -120.3585804411932116, 78.81711354060604435 ) ) ;
#8309=LINE ( 'NONE', #18070, #6538 ) ;
#8324=AXIS2_PLACEMENT_3D ( 'NONE', #15067, #860, #10402 ) ;
#8327=DIRECTION ( 'NONE',  ( -1.000000000000000000, 0.000000000000000000, 0.000000000000000000 ) ) ;
#8330=EDGE_CURVE ( 'NONE', #10075, #13187, #7286, .T. ) ;
#8341=DIRECTION ( 'NONE',  ( 0.000000000000000000, 0.000000000000000000, -1.000000000000000000 ) ) ;
#8350=CARTESIAN_POINT ( 'NONE',  ( 30.45951780490842964, -42.11129053589831273, 66.34974750395082310 ) ) ;
#8355=CARTESIAN_POINT ( 'NONE',  ( 30.00000000000000000, -85.00000000000000000, -1.040949779275250179E-14 ) ) ;
#8365=DIRECTION ( 'NONE',  ( 1.000000000000000000, 0.000000000000000000, 0.000000000000000000 ) ) ;
#8367=EDGE_CURVE ( 'NONE', #19655, #20282, #13613, .T. ) ;
#8375=CARTESIAN_POINT ( 'NONE',  ( 30.00000000000000000, -85.00000000000000000, 44.99999999999999289 ) ) ;
#8377=CARTESIAN_POINT ( 'NONE',  ( -30.00000000000000000, -164.9999999999999716, -90.00000000000001421 ) ) ;
#8378=ORIENTED_EDGE ( 'NONE', *, *, #9777, .F. ) ;
#8382=CARTESIAN_POINT ( 'NONE',  ( 31.53841889410551858, -36.05911901809099618, -66.76397724368483466 ) ) ;
#8385=LINE ( 'NONE', #14856, #12753 ) ;
#8386=B_SPLINE_CURVE_WITH_KNOTS ( 'NONE', 3,
 ( #17970, #13417, #161, #6614, #11401, #3342, #12131, #11812, #13614, #20387, #11907, #8627, #15203, #8736, #18491, #2173, #902, #5656, #2595, #15304, #589, #17000, #13516, #18275, #792, #20277, #19959, #9063, #7240, #3852, #20172, #10541, #10657, #2377, #2277, #15516, #7453, #8830, #12231, #5438, #3740, #4176, #13934, #17112, #7131, #13723, #3958, #7353, #5546, #18383, #5756, #7038, #10222, #20062, #13833, #10439, #682, #18598, #12022, #16901, #10328, #16684 ),
 .UNSPECIFIED., .F., .F.,
 ( 4, 2, 2, 2, 2, 2, 2, 2, 2, 2, 2, 2, 2, 2, 2, 2, 2, 2, 2, 2, 2, 2, 2, 2, 2, 2, 2, 2, 2, 2, 4 ),
 ( 4.770489558936219510E-18, 0.004535346501671356362, 0.009070693003342707519, 0.01020452962876053533, 0.01133836625417836662, 0.01360603950501402398, 0.01814138600668536994, 0.02040905925752104291, 0.02267673250835672283, 0.02494440575919239581, 0.02607824238461022362, 0.02721207901002805490, 0.03174742551169939392, 0.03401509876253507036, 0.03628277201337073987, 0.03855044526420640938, 0.03968428188962424413, 0.04081811851504207889, 0.04535346501671341790, 0.04648730164213123878, 0.04762113826754905965, 0.04988881151838471528, 0.05215648476922036397, 0.05329032139463818485, 0.05442415802005600572, 0.05895950452172729617, 0.06122717777256291710, 0.06349485102339853804, 0.06576252427423416591, 0.06803019752506979378, 0.07256554402674104953 ),
 .UNSPECIFIED. ) ;
#8390=ORIENTED_EDGE ( 'NONE', *, *, #11328, .T. ) ;
#8392=CARTESIAN_POINT ( 'NONE',  ( 33.27784500038035276, -116.0044176110160805, -81.92767505305181430 ) ) ;
#8397=ORIENTED_EDGE ( 'NONE', *, *, #15850, .T. ) ;
#8401=DIRECTION ( 'NONE',  ( 0.000000000000000000, 0.000000000000000000, -1.000000000000000000 ) ) ;
#8403=LINE ( 'NONE', #12788, #5178 ) ;
#8407=ORIENTED_EDGE ( 'NONE', *, *, #8433, .F. ) ;
#8410=CARTESIAN_POINT ( 'NONE',  ( 10.00000000000000178, -164.9999999999999716, 70.00000000000000000 ) ) ;
#8413=FACE_OUTER_BOUND ( 'NONE', #20695, .T. ) ;
#8414=DIRECTION ( 'NONE',  ( -1.000000000000000000, 0.000000000000000000, 0.000000000000000000 ) ) ;
#8416=CARTESIAN_POINT ( 'NONE',  ( 21.45900938229203447, -1.326995226329893862, 84.99999999999998579 ) ) ;
#8419=EDGE_CURVE ( 'NONE', #5793, #19712, #9201, .T. ) ;
#8422=CYLINDRICAL_SURFACE ( 'NONE', #5973, 40.00000000000000000 ) ;
#8423=ORIENTED_EDGE ( 'NONE', *, *, #15552, .T. ) ;
#8425=EDGE_CURVE ( 'NONE', #20805, #11718, #839, .T. ) ;
#8433=EDGE_CURVE ( 'NONE', #6575, #5439, #7394, .T. ) ;
#8439=AXIS2_PLACEMENT_3D ( 'NONE', #14497, #2932, #17569 ) ;
#8445=ADVANCED_FACE ( 'NONE', ( #952 ), #10374, .T. ) ;
#8446=CARTESIAN_POINT ( 'NONE',  ( -30.00000000000000000, -30.00000000000000000, -120.0000000000000142 ) ) ;
#8447=CARTESIAN_POINT ( 'NONE',  ( 40.61263533699685979, -122.6742132524189799, -80.56091063035071898 ) ) ;
#8448=ORIENTED_EDGE ( 'NONE', *, *, #6727, .T. ) ;
#8450=ORIENTED_EDGE ( 'NONE', *, *, #6254, .T. ) ;
#8451=FACE_OUTER_BOUND ( 'NONE', #7954, .T. ) ;
#8455=DIRECTION ( 'NONE',  ( 1.000000000000000000, 0.000000000000000000, 0.000000000000000000 ) ) ;
#8467=VECTOR ( 'NONE', #13581, 1000.000000000000000 ) ;
#8475=CARTESIAN_POINT ( 'NONE',  ( 35.04712401412363221, -25.07488921081336031, 74.50762343122646314 ) ) ;
#8477=EDGE_LOOP ( 'NONE', ( #14290, #11040, #4354, #1658, #3736 ) ) ;
#8480=CARTESIAN_POINT ( 'NONE',  ( -30.00000000000000000, -164.9999999999999716, -90.00000000000001421 ) ) ;
#8484=CARTESIAN_POINT ( 'NONE',  ( 29.99999999999999289, -105.9516309319580927, -77.66854791982075312 ) ) ;
#8485=CIRCLE ( 'NONE', #11214, 75.00000000000000000 ) ;
#8490=LINE ( 'NONE', #16658, #18330 ) ;
#8494=CIRCLE ( 'NONE', #5453, 54.99999999999999289 ) ;
#8495=VERTEX_POINT ( 'NONE', #19264 ) ;
#8498=ORIENTED_EDGE ( 'NONE', *, *, #7537, .T. ) ;
#8500=LINE ( 'NONE', #17576, #11761 ) ;
#8501=EDGE_CURVE ( 'NONE', #15340, #834, #9562, .T. ) ;
#8509=VECTOR ( 'NONE', #15977, 1000.000000000000000 ) ;
#8517=AXIS2_PLACEMENT_3D ( 'NONE', #12109, #8920, #1310 ) ;
#8518=ORIENTED_EDGE ( 'NONE', *, *, #17015, .F. ) ;
#8520=DIRECTION ( 'NONE',  ( 0.000000000000000000, 0.000000000000000000, -1.000000000000000000 ) ) ;
#8523=PLANE ( 'NONE',  #14498 ) ;
#8524=VERTEX_POINT ( 'NONE', #1274 ) ;
#8525=DIRECTION ( 'NONE',  ( 0.000000000000000000, 0.000000000000000000, -1.000000000000000000 ) ) ;
#8527=CARTESIAN_POINT ( 'NONE',  ( 30.00000000000000000, -42.57363661491096707, -121.3828884801879155 ) ) ;
#8530=AXIS2_PLACEMENT_3D ( 'NONE', #3085, #6266, #1406 ) ;
#8531=AXIS2_PLACEMENT_3D ( 'NONE', #9638, #11432, #1688 ) ;
#8543=LINE ( 'NONE', #13853, #47 ) ;
#8548=CARTESIAN_POINT ( 'NONE',  ( 39.26462282368914458, -121.8800016488677045, 86.53530536249577665 ) ) ;
#8551=B_SPLINE_CURVE_WITH_KNOTS ( 'NONE', 3,
 ( #1721, #8174, #6579, #3499, #8382, #14853, #5002, #11467, #17072, #8787, #5714, #16641, #18655, #20018, #7091, #13572, #6994, #5610 ),
 .UNSPECIFIED., .F., .F.,
 ( 4, 2, 2, 2, 2, 2, 2, 2, 4 ),
 ( 0.007425583459339141733, 0.01237513299207264328, 0.01484990775843938321, 0.01732468252480612314, 0.02722378159027312797, 0.02969855635663987137, 0.03217333112300661130, 0.03712288065574009810, 0.04702197972120707170 ),
 .UNSPECIFIED. ) ;
#8552=ORIENTED_EDGE ( 'NONE', *, *, #15380, .F. ) ;
#8554=ORIENTED_EDGE ( 'NONE', *, *, #8676, .T. ) ;
#8558=ORIENTED_EDGE ( 'NONE', *, *, #14886, .T. ) ;
#8559=LINE ( 'NONE', #5380, #8018 ) ;
#8561=EDGE_CURVE ( 'NONE', #14529, #13850, #1681, .T. ) ;
#8564=DIRECTION ( 'NONE',  ( 1.000000000000000000, -0.000000000000000000, -0.000000000000000000 ) ) ;
#8569=DIRECTION ( 'NONE',  ( 1.000000000000000000, 0.000000000000000000, 0.000000000000000000 ) ) ;
#8573=AXIS2_PLACEMENT_3D ( 'NONE', #342, #3110, #13279 ) ;
#8581=CYLINDRICAL_SURFACE ( 'NONE', #3530, 49.99999999999998579 ) ;
#8585=DIRECTION ( 'NONE',  ( 0.000000000000000000, 0.000000000000000000, -1.000000000000000000 ) ) ;
#8592=DIRECTION ( 'NONE',  ( 0.000000000000000000, 0.000000000000000000, -1.000000000000000000 ) ) ;
#8595=LINE ( 'NONE', #15379, #13999 ) ;
#8600=DIRECTION ( 'NONE',  ( 1.000000000000000000, -0.000000000000000000, -0.000000000000000000 ) ) ;
#8601=( NAMED_UNIT ( * ) SI_UNIT ( $, .STERADIAN. ) SOLID_ANGLE_UNIT ( ) );
#8608=CARTESIAN_POINT ( 'NONE',  ( -1.588862400715390422, -21.45483734977870327, 70.59898835680728268 ) ) ;
#8609=EDGE_LOOP ( 'NONE', ( #3706, #3881, #7146, #16800 ) ) ;
#8627=CARTESIAN_POINT ( 'NONE',  ( -17.67520963998171268, -12.31071423659304109, -75.43714694428801693 ) ) ;
#8647=FACE_OUTER_BOUND ( 'NONE', #18624, .T. ) ;
#8654=ORIENTED_EDGE ( 'NONE', *, *, #16553, .T. ) ;
#8662=B_SPLINE_CURVE_WITH_KNOTS ( 'NONE', 3,
 ( #17091, #20146, #13397, #8716, #5635, #4148, #14978, #12112, #20038, #7219, #19845, #15184, #16661, #3827, #12209, #15278, #18580, #5522, #5324, #2151, #18468, #8923, #18677, #11792, #10632, #13497, #8806, #8608, #18255, #2574, #7110, #15081, #7017, #7330, #19939, #4040, #15392, #10517, #10312, #661, #16974, #13590, #876, #13815, #20259, #5736, #9349, #10937, #15709, #13913, #4260, #20582, #9453, #2994, #15814, #17417, #15913, #1409, #1313, #17523, #20362, #10834 ),
 .UNSPECIFIED., .F., .F.,
 ( 4, 2, 2, 2, 2, 2, 2, 2, 2, 2, 2, 2, 2, 2, 2, 2, 2, 2, 2, 2, 2, 2, 2, 2, 2, 2, 2, 2, 2, 2, 4 ),
 ( 2.168404344971008868E-18, 0.004535346501671345953, 0.009070693003342690172, 0.01020452962876052493, 0.01133836625417835621, 0.01360603950501402572, 0.01814138600668535259, 0.02040905925752101516, 0.02267673250835667773, 0.02494440575919234376, 0.02607824238461017852, 0.02721207901002800980, 0.03174742551169934535, 0.03401509876253500098, 0.03628277201337066354, 0.03855044526420633999, 0.03968428188962416781, 0.04081811851504199562, 0.04535346501671329994, 0.04648730164213112082, 0.04762113826754894169, 0.04988881151838459038, 0.05215648476922023907, 0.05329032139463805995, 0.05442415802005587389, 0.05895950452172714351, 0.06122717777256279220, 0.06349485102339844089, 0.06576252427423409652, 0.06803019752506973827, 0.07256554402674102178 ),
 .UNSPECIFIED. ) ;
#8673=CARTESIAN_POINT ( 'NONE',  ( -30.00000000000000000, -42.57363661491096707, 121.3828884801879155 ) ) ;
#8676=EDGE_CURVE ( 'NONE', #11554, #9763, #3019, .T. ) ;
#8678=CYLINDRICAL_SURFACE ( 'NONE', #6666, 75.00000000000000000 ) ;
#8679=DIRECTION ( 'NONE',  ( 1.000000000000000000, 0.000000000000000000, 0.000000000000000000 ) ) ;
#8681=EDGE_LOOP ( 'NONE', ( #5822, #801, #11916, #14768, #3725, #11533, #13025, #9964 ) ) ;
#8688=CYLINDRICAL_SURFACE ( 'NONE', #12946, 54.99999999999999289 ) ;
#8689=AXIS2_PLACEMENT_3D ( 'NONE', #6958, #7165, #19896 ) ;
#8690=ORIENTED_EDGE ( 'NONE', *, *, #1444, .F. ) ;
#8695=EDGE_LOOP ( 'NONE', ( #12892, #549, #10815, #17809, #9893 ) ) ;
#8699=DIRECTION ( 'NONE',  ( 0.000000000000000000, -0.000000000000000000, -1.000000000000000000 ) ) ;
#8700=AXIS2_PLACEMENT_3D ( 'NONE', #8527, #5670, #604 ) ;
#8701=DIRECTION ( 'NONE',  ( 1.000000000000000000, 0.000000000000000000, 0.000000000000000000 ) ) ;
#8703=AXIS2_PLACEMENT_3D ( 'NONE', #7295, #18547, #12284 ) ;
#8707=PRESENTATION_STYLE_ASSIGNMENT (( #13176 ) ) ;
#8709=CARTESIAN_POINT ( 'NONE',  ( 30.00000000000000000, -29.99999999999999645, -45.00000000000000000 ) ) ;
#8711=ORIENTED_EDGE ( 'NONE', *, *, #16603, .T. ) ;
#8714=VERTEX_POINT ( 'NONE', #3356 ) ;
#8716=CARTESIAN_POINT ( 'NONE',  ( -20.80121494421294415, -5.547499958777468265, 80.68520720011532887 ) ) ;
#8720=ORIENTED_EDGE ( 'NONE', *, *, #14277, .F. ) ;
#8723=DIRECTION ( 'NONE',  ( -1.000000000000000000, 0.000000000000000000, 0.000000000000000000 ) ) ;
#8726=ORIENTED_EDGE ( 'NONE', *, *, #8885, .T. ) ;
#8732=ORIENTED_EDGE ( 'NONE', *, *, #16961, .T. ) ;
#8736=CARTESIAN_POINT ( 'NONE',  ( -15.44968093174340140, -14.96845338175448781, -73.80849194119340950 ) ) ;
#8747=EDGE_CURVE ( 'NONE', #20075, #13834, #13433, .T. ) ;
#8753=ORIENTED_EDGE ( 'NONE', *, *, #4751, .T. ) ;
#8763=ORIENTED_EDGE ( 'NONE', *, *, #17082, .T. ) ;
#8764=LINE ( 'NONE', #12060, #13946 ) ;
#8770=DIRECTION ( 'NONE',  ( 0.000000000000000000, 0.000000000000000000, -1.000000000000000000 ) ) ;
#8771=CARTESIAN_POINT ( 'NONE',  ( 0.000000000000000000, 0.000000000000000000, 68.00000000000000000 ) ) ;
#8783=VERTEX_POINT ( 'NONE', #18093 ) ;
#8787=CARTESIAN_POINT ( 'NONE',  ( 35.95678405163886282, -23.08991427661194606, -69.94389397731961822 ) ) ;
#8791=CARTESIAN_POINT ( 'NONE',  ( 50.00000000000000000, -164.9999999999999716, 90.00000000000001421 ) ) ;
#8798=EDGE_CURVE ( 'NONE', #9320, #2408, #18717, .T. ) ;
#8801=DIRECTION ( 'NONE',  ( 1.000000000000000000, 0.000000000000000000, 0.000000000000000000 ) ) ;
#8802=VERTEX_POINT ( 'NONE', #17894 ) ;
#8803=DIRECTION ( 'NONE',  ( 0.000000000000000000, 1.000000000000000000, 1.541976423090495387E-16 ) ) ;
#8806=CARTESIAN_POINT ( 'NONE',  ( -3.108800563652534432, -21.28778730843814060, 70.66877985699922249 ) ) ;
#8807=AXIS2_PLACEMENT_3D ( 'NONE', #18061, #3527, #14983 ) ;
#8809=DIRECTION ( 'NONE',  ( 0.000000000000000000, -1.541976423090495387E-16, 1.000000000000000000 ) ) ;
#8810=ORIENTED_EDGE ( 'NONE', *, *, #19834, .T. ) ;
#8816=ADVANCED_FACE ( 'NONE', ( #3558 ), #8229, .T. ) ;
#8819=CARTESIAN_POINT ( 'NONE',  ( 30.00000000000000000, -47.50729195424787576, -66.54687817268471406 ) ) ;
#8821=EDGE_CURVE ( 'NONE', #5556, #10438, #14647, .T. ) ;
#8829=VERTEX_POINT ( 'NONE', #13633 ) ;
#8830=CARTESIAN_POINT ( 'NONE',  ( 9.140901424055394742, -19.46372757881361792, -71.47335990888088020 ) ) ;
#8831=ORIENTED_EDGE ( 'NONE', *, *, #2561, .T. ) ;
#8833=DIRECTION ( 'NONE',  ( -1.000000000000000000, 0.000000000000000000, 0.000000000000000000 ) ) ;
#8836=ORIENTED_EDGE ( 'NONE', *, *, #2211, .T. ) ;
#8837=AXIS2_PLACEMENT_3D ( 'NONE', #9476, #16352, #9581 ) ;
#8843=ORIENTED_EDGE ( 'NONE', *, *, #1359, .F. ) ;
#8844=CARTESIAN_POINT ( 'NONE',  ( 0.000000000000000000, 0.000000000000000000, 68.00000000000000000 ) ) ;
#8849=EDGE_CURVE ( 'NONE', #20286, #19852, #17017, .T. ) ;
#8850=CARTESIAN_POINT ( 'NONE',  ( 24.99999999999999645, -99.99999999999998579, 52.00000000000000000 ) ) ;
#8855=EDGE_LOOP ( 'NONE', ( #10579, #17597 ) ) ;
#8858=ORIENTED_EDGE ( 'NONE', *, *, #4880, .T. ) ;
#8861=DIRECTION ( 'NONE',  ( -1.000000000000000000, 0.000000000000000000, 0.000000000000000000 ) ) ;
#8863=CARTESIAN_POINT ( 'NONE',  ( 33.76967208201212145, -116.6944083555470826, 82.37802687633472942 ) ) ;
#8867=CARTESIAN_POINT ( 'NONE',  ( 3.868535272439428407, -22.67561597872231616, -75.51271470091462845 ) ) ;
#8874=VERTEX_POINT ( 'NONE', #20406 ) ;
#8885=EDGE_CURVE ( 'NONE', #10995, #10075, #442, .T. ) ;
#8896=FACE_BOUND ( 'NONE', #14505, .T. ) ;
#8897=ORIENTED_EDGE ( 'NONE', *, *, #6796, .T. ) ;
#8900=DIRECTION ( 'NONE',  ( 0.000000000000000000, 0.000000000000000000, -1.000000000000000000 ) ) ;
#8901=DIRECTION ( 'NONE',  ( 1.000000000000000000, 0.000000000000000000, -0.000000000000000000 ) ) ;
#8904=CARTESIAN_POINT ( 'NONE',  ( -8.500000000000000000, 1.040949779275250140E-15, 90.00000000000000000 ) ) ;
#8908=CARTESIAN_POINT ( 'NONE',  ( -18.00000000000000000, 2.204364238465235428E-15, -130.0000000000000000 ) ) ;
#8911=CIRCLE ( 'NONE', #13314, 50.00000000000001421 ) ;
#8913=ADVANCED_FACE ( 'NONE', ( #699 ), #20192, .F. ) ;
#8914=CARTESIAN_POINT ( 'NONE',  ( 93.70999227554992217, -50.00000000000000000, -90.00000000000001421 ) ) ;
#8916=CARTESIAN_POINT ( 'NONE',  ( 50.00000000000000000, -105.0000000000000000, -90.00000000000001421 ) ) ;
#8917=DIRECTION ( 'NONE',  ( 1.000000000000000000, -0.000000000000000000, -0.000000000000000000 ) ) ;
#8918=CIRCLE ( 'NONE', #16365, 2.099999999999997868 ) ;
#8920=DIRECTION ( 'NONE',  ( -1.000000000000000000, -0.000000000000000000, -0.000000000000000000 ) ) ;
#8923=CARTESIAN_POINT ( 'NONE',  ( -9.587454675490707956, -19.24766271911509463, 71.57389447320451836 ) ) ;
#8929=CARTESIAN_POINT ( 'NONE',  ( 19.74873734152915716, 24.74873734152916072, -130.0000000000000000 ) ) ;
#8931=AXIS2_PLACEMENT_3D ( 'NONE', #1840, #17641, #246 ) ;
#8940=CIRCLE ( 'NONE', #12683, 11.50000000000000000 ) ;
#8948=DIRECTION ( 'NONE',  ( 0.000000000000000000, 0.000000000000000000, 1.000000000000000000 ) ) ;
#8949=ORIENTED_EDGE ( 'NONE', *, *, #4275, .T. ) ;
#8953=VERTEX_POINT ( 'NONE', #19975 ) ;
#8963=LINE ( 'NONE', #1021, #7355 ) ;
#8968=ORIENTED_EDGE ( 'NONE', *, *, #17139, .F. ) ;
#8971=ADVANCED_FACE ( 'NONE', ( #3975 ), #4075, .F. ) ;
#8980=FACE_OUTER_BOUND ( 'NONE', #16978, .T. ) ;
#8982=CARTESIAN_POINT ( 'NONE',  ( 0.8121682023710344867, -22.99840189857037842, -75.37408292472038340 ) ) ;
#8989=CARTESIAN_POINT ( 'NONE',  ( 45.93925756638552116, -7.831954179031021646, -85.40612192029891503 ) ) ;
#8992=DIRECTION ( 'NONE',  ( 1.000000000000000000, -0.000000000000000000, -0.000000000000000000 ) ) ;
#8998=B_SPLINE_CURVE_WITH_KNOTS ( 'NONE', 3,
 ( #15509, #9258, #5861, #12335, #18802, #15720 ),
 .UNSPECIFIED., .F., .F.,
 ( 4, 2, 4 ),
 ( 1.734723475976807094E-18, 0.003996741055817019245, 0.007993482111634036755 ),
 .UNSPECIFIED. ) ;
#9001=CARTESIAN_POINT ( 'NONE',  ( 45.22159793441013420, -8.673994507468389514, -84.62946326583126222 ) ) ;
#9016=AXIS2_PLACEMENT_3D ( 'NONE', #13896, #7312, #12097 ) ;
#9018=B_SPLINE_CURVE_WITH_KNOTS ( 'NONE', 3,
 ( #6252, #4979, #14932, #6861, #16115, #408, #6664, #6450 ),
 .UNSPECIFIED., .F., .F.,
 ( 4, 2, 2, 4 ),
 ( 1.734723475976807094E-18, 0.005430084938242705703, 0.008145127407364069830, 0.01086016987648543569 ),
 .UNSPECIFIED. ) ;
#9024=FACE_OUTER_BOUND ( 'NONE', #3111, .T. ) ;
#9029=AXIS2_PLACEMENT_3D ( 'NONE', #14428, #1299, #9124 ) ;
#9030=DIRECTION ( 'NONE',  ( 0.000000000000000000, -1.000000000000000000, 0.000000000000000000 ) ) ;
#9042=ORIENTED_EDGE ( 'NONE', *, *, #10981, .T. ) ;
#9043=EDGE_CURVE ( 'NONE', #6265, #10714, #3478, .T. ) ;
#9050=VECTOR ( 'NONE', #7049, 1000.000000000000000 ) ;
#9058=ORIENTED_EDGE ( 'NONE', *, *, #26, .T. ) ;
#9063=CARTESIAN_POINT ( 'NONE',  ( -1.588862400715383316, -21.45483734977869261, -70.59898835680725426 ) ) ;
#9068=CARTESIAN_POINT ( 'NONE',  ( -30.00000000000000000, 29.99999999999999289, -120.0000000000000142 ) ) ;
#9076=FACE_OUTER_BOUND ( 'NONE', #4020, .T. ) ;
#9078=SHAPE_DEFINITION_REPRESENTATION ( #3557, #4392 ) ;
#9084=EDGE_LOOP ( 'NONE', ( #11175, #15097, #11446, #12618 ) ) ;
#9085=DIRECTION ( 'NONE',  ( 0.000000000000000000, 3.469446951953615175E-16, 1.000000000000000000 ) ) ;
#9088=DIRECTION ( 'NONE',  ( 1.000000000000000000, -0.000000000000000000, -0.000000000000000000 ) ) ;
#9090=ORIENTED_EDGE ( 'NONE', *, *, #9606, .F. ) ;
#9094=DIRECTION ( 'NONE',  ( 1.000000000000000000, -0.000000000000000000, -0.000000000000000000 ) ) ;
#9100=EDGE_CURVE ( 'NONE', #3970, #11744, #4821, .T. ) ;
#9106=EDGE_CURVE ( 'NONE', #19457, #13026, #1135, .T. ) ;
#9108=ORIENTED_EDGE ( 'NONE', *, *, #15798, .T. ) ;
#9109=CARTESIAN_POINT ( 'NONE',  ( 24.99999999999999645, -39.99999999999999289, -54.09999999999999432 ) ) ;
#9122=ORIENTED_EDGE ( 'NONE', *, *, #5809, .T. ) ;
#9124=DIRECTION ( 'NONE',  ( 0.000000000000000000, 0.000000000000000000, 1.000000000000000000 ) ) ;
#9137=ORIENTED_EDGE ( 'NONE', *, *, #14530, .F. ) ;
#9145=DIRECTION ( 'NONE',  ( 1.000000000000000000, 0.000000000000000000, 0.000000000000000000 ) ) ;
#9147=EDGE_LOOP ( 'NONE', ( #13185, #3574, #18650, #458 ) ) ;
#9167=ORIENTED_EDGE ( 'NONE', *, *, #9338, .T. ) ;
#9171=CIRCLE ( 'NONE', #7121, 8.999999999999994671 ) ;
#9172=EDGE_LOOP ( 'NONE', ( #5547, #830 ) ) ;
#9181=CARTESIAN_POINT ( 'NONE',  ( 14.14403058282573689, -16.24569260159238837, 78.86174789526529594 ) ) ;
#9184=LINE ( 'NONE', #7912, #16964 ) ;
#9187=ORIENTED_EDGE ( 'NONE', *, *, #1614, .T. ) ;
#9189=DIRECTION ( 'NONE',  ( 1.000000000000000000, -0.000000000000000000, -0.000000000000000000 ) ) ;
#9193=CARTESIAN_POINT ( 'NONE',  ( 20.21512691275406937, -10.97478183557446307, -82.63187968860285082 ) ) ;
#9196=VERTEX_POINT ( 'NONE', #3336 ) ;
#9198=AXIS2_PLACEMENT_3D ( 'NONE', #10831, #12321, #2455 ) ;
#9201=LINE ( 'NONE', #12167, #13285 ) ;
#9206=EDGE_CURVE ( 'NONE', #9763, #5350, #9702, .T. ) ;
#9213=ORIENTED_EDGE ( 'NONE', *, *, #17105, .T. ) ;
#9214=CARTESIAN_POINT ( 'NONE',  ( -31.35784117651625635, 26.35784117651607872, -120.0000000000000142 ) ) ;
#9219=EDGE_CURVE ( 'NONE', #15337, #3206, #20056, .T. ) ;
#9220=DIRECTION ( 'NONE',  ( 0.000000000000000000, 0.000000000000000000, -1.000000000000000000 ) ) ;
#9222=CARTESIAN_POINT ( 'NONE',  ( 0.000000000000000000, 0.000000000000000000, -90.00000000000000000 ) ) ;
#9224=EDGE_CURVE ( 'NONE', #15415, #5413, #8309, .T. ) ;
#9227=CARTESIAN_POINT ( 'NONE',  ( 33.68763977253520636, -116.6032510994795217, -76.49582849428456655 ) ) ;
#9233=AXIS2_PLACEMENT_3D ( 'NONE', #3147, #9812, #7717 ) ;
#9235=LINE ( 'NONE', #12313, #13933 ) ;
#9238=PLANE ( 'NONE',  #16140 ) ;
#9252=CARTESIAN_POINT ( 'NONE',  ( 30.43430782549247837, -42.57363661491096707, -71.38288848018790134 ) ) ;
#9253=DIRECTION ( 'NONE',  ( 0.000000000000000000, 0.000000000000000000, 1.000000000000000000 ) ) ;
#9254=EDGE_CURVE ( 'NONE', #16423, #16359, #19070, .T. ) ;
#9258=CARTESIAN_POINT ( 'NONE',  ( 45.93925756638542879, -7.831954179031023422, 85.40612192029894345 ) ) ;
#9269=CARTESIAN_POINT ( 'NONE',  ( 23.13963350654227824, -26.35784117651622793, -120.0000000000000142 ) ) ;
#9277=CIRCLE ( 'NONE', #3505, 75.00000000000000000 ) ;
#9284=CARTESIAN_POINT ( 'NONE',  ( 30.98133542675971341, -111.2038170487246447, 74.06521627071094827 ) ) ;
#9285=EDGE_CURVE ( 'NONE', #4186, #4931, #12304, .T. ) ;
#9301=CARTESIAN_POINT ( 'NONE',  ( 9.663423836078200324, -20.87488706538416139, -76.33627221503081728 ) ) ;
#9313=VERTEX_POINT ( 'NONE', #2053 ) ;
#9318=B_SPLINE_CURVE_WITH_KNOTS ( 'NONE', 3,
 ( #19515, #123, #5093, #8084, #16540, #6685, #14553, #14749, #8475, #16139, #438, #20, #11254, #229, #12860, #11559, #19303, #9672, #17936, #9865, #1824, #17733 ),
 .UNSPECIFIED., .F., .F.,
 ( 4, 2, 2, 2, 2, 2, 2, 2, 2, 2, 4 ),
 ( 0.008732568481177037031, 0.01468344170611684228, 0.02063431493105664927, 0.02658518815599645452, 0.03253606138093625977, 0.03551149799340617974, 0.03848693460587609277, 0.04443780783081591884, 0.05038868105575574491, 0.05336411766822565100, 0.05633955428069555710 ),
 .UNSPECIFIED. ) ;
#9320=VERTEX_POINT ( 'NONE', #17961 ) ;
#9323=FACE_OUTER_BOUND ( 'NONE', #19401, .T. ) ;
#9326=ORIENTED_EDGE ( 'NONE', *, *, #2056, .F. ) ;
#9329=ORIENTED_EDGE ( 'NONE', *, *, #18690, .T. ) ;
#9331=CARTESIAN_POINT ( 'NONE',  ( 38.17990591115487575, -121.1390473681899351, -79.37944074850724974 ) ) ;
#9332=VECTOR ( 'NONE', #1214, 1000.000000000000000 ) ;
#9334=DIRECTION ( 'NONE',  ( 1.000000000000000000, 0.000000000000000000, -0.000000000000000000 ) ) ;
#9338=EDGE_CURVE ( 'NONE', #19615, #20567, #17032, .T. ) ;
#9343=DIRECTION ( 'NONE',  ( -0.000000000000000000, -0.000000000000000000, 1.000000000000000000 ) ) ;
#9344=ORIENTED_EDGE ( 'NONE', *, *, #6504, .T. ) ;
#9345=CARTESIAN_POINT ( 'NONE',  ( 24.99999999999999645, -85.00000000000000000, -1.040949779275250179E-14 ) ) ;
#9349=CARTESIAN_POINT ( 'NONE',  ( 14.87228507261736432, -15.53036221685708362, 73.48983352790762069 ) ) ;
#9357=FACE_OUTER_BOUND ( 'NONE', #19314, .T. ) ;
#9358=DIRECTION ( 'NONE',  ( -1.000000000000000000, -0.000000000000000000, -0.000000000000000000 ) ) ;
#9362=DIRECTION ( 'NONE',  ( 0.000000000000000000, 0.000000000000000000, -1.000000000000000000 ) ) ;
#9374=EDGE_CURVE ( 'NONE', #5793, #11740, #6867, .T. ) ;
#9376=VERTEX_POINT ( 'NONE', #15295 ) ;
#9377=LINE ( 'NONE', #20697, #2022 ) ;
#9384=DIRECTION ( 'NONE',  ( 1.000000000000000000, 0.000000000000000000, 0.000000000000000000 ) ) ;
#9389=AXIS2_PLACEMENT_3D ( 'NONE', #8033, #3450, #16500 ) ;
#9393=DIRECTION ( 'NONE',  ( -0.000000000000000000, -0.000000000000000000, 1.000000000000000000 ) ) ;
#9399=LINE ( 'NONE', #2539, #20121 ) ;
#9403=CARTESIAN_POINT ( 'NONE',  ( 19.82535189207093040, -8.394204402731995529, 84.86463929178358967 ) ) ;
#9404=AXIS2_PLACEMENT_3D ( 'NONE', #14304, #3264, #2960 ) ;
#9407=ORIENTED_EDGE ( 'NONE', *, *, #2649, .F. ) ;
#9410=CARTESIAN_POINT ( 'NONE',  ( 50.00000000000000000, -159.9999999999999716, -53.99496054166690584 ) ) ;
#9413=CARTESIAN_POINT ( 'NONE',  ( -22.55329027477439041, -4.616075264032610370, -88.80073566248103134 ) ) ;
#9414=CARTESIAN_POINT ( 'NONE',  ( 56.98610214956094211, -164.9999999999999716, 84.54208835637712127 ) ) ;
#9420=FACE_OUTER_BOUND ( 'NONE', #6030, .T. ) ;
#9425=ORIENTED_EDGE ( 'NONE', *, *, #2056, .T. ) ;
#9428=CARTESIAN_POINT ( 'NONE',  ( 50.00000000000000000, -164.9999999999999716, 90.00000000000001421 ) ) ;
#9432=DIRECTION ( 'NONE',  ( -1.000000000000000000, -0.000000000000000000, -0.000000000000000000 ) ) ;
#9434=VERTEX_POINT ( 'NONE', #4168 ) ;
#9451=VERTEX_POINT ( 'NONE', #3734 ) ;
#9453=CARTESIAN_POINT ( 'NONE',  ( 18.97564634267267181, -10.12806126886903613, 76.96678999104570096 ) ) ;
#9465=CARTESIAN_POINT ( 'NONE',  ( 0.000000000000000000, 0.000000000000000000, -90.00000000000000000 ) ) ;
#9466=CARTESIAN_POINT ( 'NONE',  ( -30.00000000000000000, 29.99999999999999289, -120.0000000000000142 ) ) ;
#9473=DIRECTION ( 'NONE',  ( 0.000000000000000000, 0.000000000000000000, -1.000000000000000000 ) ) ;
#9476=CARTESIAN_POINT ( 'NONE',  ( -30.00000000000000000, 29.99999999999999289, -130.0000000000000000 ) ) ;
#9493=CARTESIAN_POINT ( 'NONE',  ( -39.99999999999999289, -40.00000000000000000, -120.0000000000000142 ) ) ;
#9495=ORIENTED_EDGE ( 'NONE', *, *, #5070, .F. ) ;
#9496=CARTESIAN_POINT ( 'NONE',  ( 16.80839512764391586, -13.42119425201006422, 80.75675983441298911 ) ) ;
#9505=VECTOR ( 'NONE', #18683, 1000.000000000000000 ) ;
#9506=ORIENTED_EDGE ( 'NONE', *, *, #16207, .F. ) ;
#9507=CARTESIAN_POINT ( 'NONE',  ( -30.00000000000000000, -85.00000000000000000, -1.040949779275250179E-14 ) ) ;
#9510=EDGE_CURVE ( 'NONE', #20241, #7282, #7985, .T. ) ;
#9513=LINE ( 'NONE', #17684, #16644 ) ;
#9525=PLANE ( 'NONE',  #18181 ) ;
#9527=CARTESIAN_POINT ( 'NONE',  ( 10.00000000000000178, -160.0000000000000000, 70.00000000000000000 ) ) ;
#9530=CARTESIAN_POINT ( 'NONE',  ( 31.95495987947095173, -34.31614948441001900, -72.06256082998474710 ) ) ;
#9533=CIRCLE ( 'NONE', #19030, 3.199999999999994404 ) ;
#9537=CARTESIAN_POINT ( 'NONE',  ( -30.00000000000000000, -42.57363661491096707, -121.3828884801879155 ) ) ;
#9539=EDGE_CURVE ( 'NONE', #17751, #3623, #5889, .T. ) ;
#9540=FACE_OUTER_BOUND ( 'NONE', #6738, .T. ) ;
#9542=AXIS2_PLACEMENT_3D ( 'NONE', #12464, #2108, #2008 ) ;
#9547=CARTESIAN_POINT ( 'NONE',  ( 48.35276434571220250, -3.649167310370820871, 90.00000000000000000 ) ) ;
#9548=DIRECTION ( 'NONE',  ( 1.000000000000000000, 0.000000000000000000, 0.000000000000000000 ) ) ;
#9555=DIRECTION ( 'NONE',  ( 0.000000000000000000, 0.000000000000000000, -1.000000000000000000 ) ) ;
#9556=ORIENTED_EDGE ( 'NONE', *, *, #14171, .T. ) ;
#9560=ORIENTED_EDGE ( 'NONE', *, *, #9106, .T. ) ;
#9562=CIRCLE ( 'NONE', #10235, 18.00000000000000000 ) ;
#9565=FACE_OUTER_BOUND ( 'NONE', #7405, .T. ) ;
#9577=ADVANCED_FACE ( 'NONE', ( #4381 ), #14358, .T. ) ;
#9581=DIRECTION ( 'NONE',  ( -1.000000000000000000, 0.000000000000000000, 0.000000000000000000 ) ) ;
#9583=DIRECTION ( 'NONE',  ( 8.673617379884035472E-17, -1.000000000000000000, 0.000000000000000000 ) ) ;
#9586=CARTESIAN_POINT ( 'NONE',  ( 50.00000000000000000, -1.326995226329880762, -84.99999999999998579 ) ) ;
#9591=AXIS2_PLACEMENT_3D ( 'NONE', #7203, #552, #13690 ) ;
#9602=CARTESIAN_POINT ( 'NONE',  ( -2.904526653654485813, -21.31518795036016201, 76.12711593406372401 ) ) ;
#9605=CIRCLE ( 'NONE', #16040, 5.000000000000000888 ) ;
#9606=EDGE_CURVE ( 'NONE', #10438, #17156, #1424, .T. ) ;
#9610=AXIS2_PLACEMENT_3D ( 'NONE', #28, #11373, #130 ) ;
#9615=PLANE ( 'NONE',  #2240 ) ;
#9617=EDGE_LOOP ( 'NONE', ( #5882, #9187, #12332, #17418 ) ) ;
#9618=CARTESIAN_POINT ( 'NONE',  ( -11.59853973546238315, -19.87550760251307835, -76.83006856037964383 ) ) ;
#9621=CIRCLE ( 'NONE', #11316, 2.099999999999990763 ) ;
#9622=ORIENTED_EDGE ( 'NONE', *, *, #9100, .T. ) ;
#9625=LINE ( 'NONE', #10112, #8509 ) ;
#9628=ADVANCED_FACE ( 'NONE', ( #1112, #12866 ), #14862, .T. ) ;
#9630=B_SPLINE_CURVE_WITH_KNOTS ( 'NONE', 3,
 ( #10303, #13387, #11679, #18247, #3513, #18147, #5512, #6790, #16549, #10092, #8392, #5409, #7102, #243, #3714, #11573, #10410, #2033, #18458, #2244, #8484, #13175 ),
 .UNSPECIFIED., .F., .F.,
 ( 4, 2, 2, 2, 2, 2, 2, 2, 2, 2, 4 ),
 ( 0.01090777686127726055, 0.01377645490973365520, 0.01664513295819005159, 0.01807947198241826800, 0.01951381100664648441, 0.02238248905510294498, 0.02525116710355940555, 0.02668550612778763237, 0.02811984515201586265, 0.03098852320047232323, 0.03385720124892877686 ),
 .UNSPECIFIED. ) ;
#9632=ORIENTED_EDGE ( 'NONE', *, *, #13950, .T. ) ;
#9638=CARTESIAN_POINT ( 'NONE',  ( 10.00000000000000178, -164.9999999999999716, 70.00000000000000000 ) ) ;
#9648=AXIS2_PLACEMENT_3D ( 'NONE', #18995, #4582, #19210 ) ;
#9649=FACE_BOUND ( 'NONE', #14420, .T. ) ;
#9650=CARTESIAN_POINT ( 'NONE',  ( 30.00000000000000000, -30.00000000000000711, -58.09475019311124555 ) ) ;
#9653=CARTESIAN_POINT ( 'NONE',  ( 45.22159793441012710, -8.673994507468377080, 78.07221698934969822 ) ) ;
#9658=CIRCLE ( 'NONE', #15741, 2.099999999999997868 ) ;
#9660=DIRECTION ( 'NONE',  ( 0.000000000000000000, 0.000000000000000000, -1.000000000000000000 ) ) ;
#9668=CYLINDRICAL_SURFACE ( 'NONE', #15052, 80.00000000000000000 ) ;
#9671=ORIENTED_EDGE ( 'NONE', *, *, #3184, .F. ) ;
#9672=CARTESIAN_POINT ( 'NONE',  ( 30.18965574827983289, -44.98719419906327488, 71.43126268043587856 ) ) ;
#9676=CARTESIAN_POINT ( 'NONE',  ( 10.00000000000000178, -164.9999999999999716, -73.20000000000000284 ) ) ;
#9679=CARTESIAN_POINT ( 'NONE',  ( -21.50000000000000000, 2.632990618166809235E-15, 84.99999999999998579 ) ) ;
#9687=CIRCLE ( 'NONE', #1573, 2.099999999999990763 ) ;
#9688=EDGE_LOOP ( 'NONE', ( #2390, #6044, #11278, #15110 ) ) ;
#9692=ORIENTED_EDGE ( 'NONE', *, *, #4006, .F. ) ;
#9696=EDGE_CURVE ( 'NONE', #4938, #12626, #12967, .T. ) ;
#9699=DIRECTION ( 'NONE',  ( 0.000000000000000000, 0.000000000000000000, 1.000000000000000000 ) ) ;
#9702=LINE ( 'NONE', #14683, #5514 ) ;
#9711=DIRECTION ( 'NONE',  ( 0.000000000000000000, -1.000000000000000000, 0.000000000000000000 ) ) ;
#9712=DIRECTION ( 'NONE',  ( -8.673617379884035472E-17, 1.000000000000000000, 0.000000000000000000 ) ) ;
#9718=CARTESIAN_POINT ( 'NONE',  ( -14.03392052762769993, -18.23657722200194087, -77.70237658995378638 ) ) ;
#9722=VERTEX_POINT ( 'NONE', #19729 ) ;
#9723=FACE_OUTER_BOUND ( 'NONE', #8477, .T. ) ;
#9725=CIRCLE ( 'NONE', #4990, 40.00000000000000000 ) ;
#9727=DIRECTION ( 'NONE',  ( 0.000000000000000000, 0.000000000000000000, -1.000000000000000000 ) ) ;
#9740=VECTOR ( 'NONE', #16890, 1000.000000000000000 ) ;
#9741=CARTESIAN_POINT ( 'NONE',  ( 0.000000000000000000, 0.000000000000000000, -90.00000000000000000 ) ) ;
#9742=CARTESIAN_POINT ( 'NONE',  ( 35.69831387705275461, -23.59893667096173431, 69.72867780164767737 ) ) ;
#9748=CARTESIAN_POINT ( 'NONE',  ( 50.00000000000000000, -139.6410161513775563, 89.99999999999998579 ) ) ;
#9752=CARTESIAN_POINT ( 'NONE',  ( 48.84346035822958498, -2.517149734616030088, 83.65074274608480209 ) ) ;
#9753=ADVANCED_FACE ( 'NONE', ( #9779, #8091 ), #3213, .F. ) ;
#9755=DIRECTION ( 'NONE',  ( -1.000000000000000000, 0.000000000000000000, 0.000000000000000000 ) ) ;
#9763=VERTEX_POINT ( 'NONE', #18041 ) ;
#9766=CARTESIAN_POINT ( 'NONE',  ( 30.00000000000000000, -39.99999999999999289, -49.90000000000000568 ) ) ;
#9768=VERTEX_POINT ( 'NONE', #9979 ) ;
#9770=CARTESIAN_POINT ( 'NONE',  ( 30.00000000000000000, 4.299168419249259188, -90.00000000000001421 ) ) ;
#9777=EDGE_CURVE ( 'NONE', #10607, #12734, #2163, .T. ) ;
#9779=FACE_BOUND ( 'NONE', #19512, .T. ) ;
#9790=ORIENTED_EDGE ( 'NONE', *, *, #15195, .T. ) ;
#9795=CARTESIAN_POINT ( 'NONE',  ( 40.00000000000000711, -122.3205080756887639, 80.28096411455982206 ) ) ;
#9805=LINE ( 'NONE', #10018, #5797 ) ;
#9809=ORIENTED_EDGE ( 'NONE', *, *, #8885, .F. ) ;
#9812=DIRECTION ( 'NONE',  ( -0.000000000000000000, -0.000000000000000000, -1.000000000000000000 ) ) ;
#9824=FACE_OUTER_BOUND ( 'NONE', #8681, .T. ) ;
#9826=FACE_OUTER_BOUND ( 'NONE', #1290, .T. ) ;
#9832=CARTESIAN_POINT ( 'NONE',  ( 41.00037741435939154, -14.03198441848082467, 74.23899123100075315 ) ) ;
#9837=CARTESIAN_POINT ( 'NONE',  ( 0.000000000000000000, 0.000000000000000000, 81.99999999999998579 ) ) ;
#9842=CARTESIAN_POINT ( 'NONE',  ( 46.19699674809955781, -7.457365076151437400, 79.04478793936081615 ) ) ;
#9855=ORIENTED_EDGE ( 'NONE', *, *, #2600, .F. ) ;
#9865=CARTESIAN_POINT ( 'NONE',  ( 30.02347015119159224, -47.99982825264939379, 71.66797303202216085 ) ) ;
#9883=VERTEX_POINT ( 'NONE', #4133 ) ;
#9888=DIRECTION ( 'NONE',  ( 1.000000000000000000, -0.000000000000000000, -0.000000000000000000 ) ) ;
#9893=ORIENTED_EDGE ( 'NONE', *, *, #16095, .F. ) ;
#9898=DIRECTION ( 'NONE',  ( -1.000000000000000000, 0.000000000000000000, 0.000000000000000000 ) ) ;
#9901=VECTOR ( 'NONE', #192, 1000.000000000000000 ) ;
#9913=ORIENTED_EDGE ( 'NONE', *, *, #3184, .T. ) ;
#9917=DIRECTION ( 'NONE',  ( 0.000000000000000000, 0.000000000000000000, 1.000000000000000000 ) ) ;
#9918=ADVANCED_FACE ( 'NONE', ( #3813 ), #20136, .F. ) ;
#9936=CARTESIAN_POINT ( 'NONE',  ( 30.73276154958900719, -40.16863665929199811, 66.40168251036186575 ) ) ;
#9944=EDGE_CURVE ( 'NONE', #16972, #7685, #5406, .T. ) ;
#9950=CARTESIAN_POINT ( 'NONE',  ( -27.96694501150314593, -24.74873734152930993, -130.0000000000000000 ) ) ;
#9951=CARTESIAN_POINT ( 'NONE',  ( -30.00000000000000000, -85.00000000000000000, -1.040949779275250179E-14 ) ) ;
#9959=AXIS2_PLACEMENT_3D ( 'NONE', #11046, #7860, #14341 ) ;
#9961=CARTESIAN_POINT ( 'NONE',  ( 50.00000000000000000, -160.0000000000000000, 0.000000000000000000 ) ) ;
#9964=ORIENTED_EDGE ( 'NONE', *, *, #19342, .T. ) ;
#9966=ORIENTED_EDGE ( 'NONE', *, *, #210, .T. ) ;
#9967=DIRECTION ( 'NONE',  ( -1.000000000000000000, 0.000000000000000000, 0.000000000000000000 ) ) ;
#9974=FILL_AREA_STYLE ('',( #11874 ) ) ;
#9977=VECTOR ( 'NONE', #1560, 1000.000000000000000 ) ;
#9979=CARTESIAN_POINT ( 'NONE',  ( 18.00000000000000000, 0.000000000000000000, -90.00000000000000000 ) ) ;
#9980=B_SPLINE_CURVE_WITH_KNOTS ( 'NONE', 3,
 ( #13860, #4212, #20425, #2636, #10886, #18848, #7486, #9193, #15653, #12487, #2833, #13969, #20307, #15762, #7602, #4089, #18741, #10688, #7276, #5909, #18950, #4324, #17149, #9301, #7169, #18529, #13651, #10793, #8867, #20100, #12158, #829, #8982, #18625, #5577, #2724, #12058, #3990, #17038, #2526, #14397, #9618, #1675, #14506, #9718, #12586, #6326, #19257, #12813, #17887, #1470, #11203, #19159, #10992, #4636, #20841, #9413, #1265 ),
 .UNSPECIFIED., .F., .F.,
 ( 4, 2, 2, 2, 2, 2, 2, 2, 2, 2, 2, 2, 2, 2, 2, 2, 2, 2, 2, 2, 2, 2, 2, 2, 2, 2, 2, 2, 4 ),
 ( 6.992893892674702526E-18, 0.004580336630963589492, 0.009160673261927172045, 0.01030575741966808373, 0.01145084157740899541, 0.01374100989289079623, 0.01603117820837259705, 0.01717626236611349486, 0.01832134652385439266, 0.02290168315481797695, 0.02519185147029977603, 0.02633693562804066690, 0.02748201978578156124, 0.03206235641674509695, 0.03320744057448597047, 0.03435252473222685093, 0.03664269304770861185, 0.03893286136319037971, 0.04122302967867213369, 0.04580336630963566247, 0.04809353462511742339, 0.05038370294059917737, 0.05267387125608093829, 0.05496403957156269227, 0.05954437620252620716, 0.06183454451800795421, 0.06412471283348972206, 0.06870504946445318839, 0.07328538609541666859 ),
 .UNSPECIFIED. ) ;
#9986=DIRECTION ( 'NONE',  ( 0.000000000000000000, 1.000000000000000000, -8.673617379884034239E-17 ) ) ;
#9988=EDGE_LOOP ( 'NONE', ( #2531, #12582 ) ) ;
#9989=DIRECTION ( 'NONE',  ( 0.000000000000000000, -0.7812527682501556603, 0.6242147964454771714 ) ) ;
#9990=ORIENTED_EDGE ( 'NONE', *, *, #7252, .T. ) ;
#10002=DIRECTION ( 'NONE',  ( 0.000000000000000000, 0.000000000000000000, -1.000000000000000000 ) ) ;
#10003=DIRECTION ( 'NONE',  ( 1.000000000000000000, 0.000000000000000000, 0.000000000000000000 ) ) ;
#10005=AXIS2_PLACEMENT_3D ( 'NONE', #16033, #4376, #20684 ) ;
#10006=ADVANCED_FACE ( 'NONE', ( #4569 ), #1192, .F. ) ;
#10007=DIRECTION ( 'NONE',  ( 1.000000000000000000, 0.000000000000000000, 0.000000000000000000 ) ) ;
#10011=CARTESIAN_POINT ( 'NONE',  ( 0.000000000000000000, 0.000000000000000000, 68.00000000000000000 ) ) ;
#10016=CARTESIAN_POINT ( 'NONE',  ( 50.00000000000000000, -97.49621075554985339, -111.6458212409894486 ) ) ;
#10017=ORIENTED_EDGE ( 'NONE', *, *, #6087, .F. ) ;
#10018=CARTESIAN_POINT ( 'NONE',  ( 50.00000000000000000, -124.9999999999999858, -90.00000000000001421 ) ) ;
#10024=DIRECTION ( 'NONE',  ( 0.000000000000000000, 0.000000000000000000, -1.000000000000000000 ) ) ;
#10025=B_SPLINE_CURVE_WITH_KNOTS ( 'NONE', 3,
 ( #20661, #7633, #17287, #14114, #9331, #2761, #2667, #14216, #10919, #9227, #1394, #4672, #12627, #4565, #16004, #20568, #6045, #20874, #19088, #12518 ),
 .UNSPECIFIED., .F., .F.,
 ( 4, 2, 2, 2, 2, 2, 2, 2, 2, 4 ),
 ( 0.01071967184985863145, 0.01211474467708338262, 0.01350981750430813380, 0.01629996315875761187, 0.01909010881320709341, 0.02188025446765657148, 0.02467040012210604955, 0.02606547294933077297, 0.02746054577655549292, 0.03304083708545443171 ),
 .UNSPECIFIED. ) ;
#10027=DIRECTION ( 'NONE',  ( 0.000000000000000000, -1.040834085586084454E-15, 1.000000000000000000 ) ) ;
#10042=FACE_BOUND ( 'NONE', #2309, .T. ) ;
#10045=EDGE_CURVE ( 'NONE', #20820, #14202, #7747, .T. ) ;
#10047=DIRECTION ( 'NONE',  ( 0.000000000000000000, 3.469446951953615175E-16, 1.000000000000000000 ) ) ;
#10048=ORIENTED_EDGE ( 'NONE', *, *, #10045, .F. ) ;
#10049=CARTESIAN_POINT ( 'NONE',  ( 38.55309439416022599, -121.4058261247164268, 86.08339649466212506 ) ) ;
#10050=CARTESIAN_POINT ( 'NONE',  ( 44.24299768761039786, -125.5422689251970638, -83.10177353372741038 ) ) ;
#10061=AXIS2_PLACEMENT_3D ( 'NONE', #7620, #4231, #6033 ) ;
#10063=LINE ( 'NONE', #19799, #5144 ) ;
#10071=AXIS2_PLACEMENT_3D ( 'NONE', #7028, #11801, #10002 ) ;
#10075=VERTEX_POINT ( 'NONE', #18892 ) ;
#10078=FACE_OUTER_BOUND ( 'NONE', #7948, .T. ) ;
#10082=LINE ( 'NONE', #228, #1074 ) ;
#10083=CARTESIAN_POINT ( 'NONE',  ( -11.50000000000000000, 0.000000000000000000, -81.99999999999998579 ) ) ;
#10088=ADVANCED_FACE ( 'NONE', ( #5943 ), #12417, .T. ) ;
#10092=CARTESIAN_POINT ( 'NONE',  ( 33.75963133984988929, -116.7035671405861308, -82.37576306755489952 ) ) ;
#10098=DIRECTION ( 'NONE',  ( -0.000000000000000000, 1.000000000000000000, 0.000000000000000000 ) ) ;
#10099=ORIENTED_EDGE ( 'NONE', *, *, #9206, .T. ) ;
#10104=DIRECTION ( 'NONE',  ( 0.000000000000000000, 0.000000000000000000, -1.000000000000000000 ) ) ;
#10107=FACE_BOUND ( 'NONE', #12757, .T. ) ;
#10110=EDGE_CURVE ( 'NONE', #13160, #19902, #19498, .T. ) ;
#10111=DIRECTION ( 'NONE',  ( 1.000000000000000000, 0.000000000000000000, 0.000000000000000000 ) ) ;
#10112=CARTESIAN_POINT ( 'NONE',  ( 50.00000000000000000, 230.0000000000000000, -85.00000000000000000 ) ) ;
#10120=ORIENTED_EDGE ( 'NONE', *, *, #7421, .F. ) ;
#10130=DIRECTION ( 'NONE',  ( 1.000000000000000000, 0.000000000000000000, 0.000000000000000000 ) ) ;
#10142=CARTESIAN_POINT ( 'NONE',  ( 0.000000000000000000, 0.000000000000000000, -130.0000000000000000 ) ) ;
#10148=ADVANCED_FACE ( 'NONE', ( #9540 ), #3382, .T. ) ;
#10167=CARTESIAN_POINT ( 'NONE',  ( 30.00000000000000000, -85.00000000000000000, -1.040949779275250179E-14 ) ) ;
#10168=CARTESIAN_POINT ( 'NONE',  ( 50.00000000000000000, -49.99999999999997868, 71.93747284969079203 ) ) ;
#10169=ORIENTED_EDGE ( 'NONE', *, *, #18089, .F. ) ;
#10173=DIRECTION ( 'NONE',  ( -1.000000000000000000, 0.000000000000000000, 0.000000000000000000 ) ) ;
#10178=CARTESIAN_POINT ( 'NONE',  ( 50.00000000000000000, 230.0000000000000000, 0.000000000000000000 ) ) ;
#10179=DIRECTION ( 'NONE',  ( -0.000000000000000000, 0.000000000000000000, -1.000000000000000000 ) ) ;
#10184=EDGE_CURVE ( 'NONE', #4685, #12559, #4795, .T. ) ;
#10187=DIRECTION ( 'NONE',  ( 0.000000000000000000, 0.000000000000000000, 1.000000000000000000 ) ) ;
#10190=CARTESIAN_POINT ( 'NONE',  ( 10.00000000000000178, -148.4917293642369600, 48.67032260359988527 ) ) ;
#10192=DIRECTION ( 'NONE',  ( -0.000000000000000000, -0.000000000000000000, 1.000000000000000000 ) ) ;
#10197=EDGE_LOOP ( 'NONE', ( #5294, #13398, #8763, #16900 ) ) ;
#10199=DIRECTION ( 'NONE',  ( 1.000000000000000000, 0.000000000000000000, 0.000000000000000000 ) ) ;
#10203=VERTEX_POINT ( 'NONE', #14941 ) ;
#10212=DIRECTION ( 'NONE',  ( -1.000000000000000000, -0.000000000000000000, -0.000000000000000000 ) ) ;
#10221=VECTOR ( 'NONE', #12031, 1000.000000000000000 ) ;
#10222=CARTESIAN_POINT ( 'NONE',  ( 18.97564634267267181, -10.12806126886902014, -76.96678999104568675 ) ) ;
#10232=CARTESIAN_POINT ( 'NONE',  ( -22.96694501150314238, -24.74873734152930993, -120.0000000000000142 ) ) ;
#10235=AXIS2_PLACEMENT_3D ( 'NONE', #12596, #9727, #4644 ) ;
#10237=CIRCLE ( 'NONE', #15991, 21.50000000000000000 ) ;
#10249=EDGE_CURVE ( 'NONE', #6577, #5841, #11854, .T. ) ;
#10254=CARTESIAN_POINT ( 'NONE',  ( 40.00000000000000000, -122.3205080756887639, 86.97287527660684248 ) ) ;
#10266=EDGE_CURVE ( 'NONE', #6177, #8249, #12709, .T. ) ;
#10281=ORIENTED_EDGE ( 'NONE', *, *, #3208, .F. ) ;
#10284=DIRECTION ( 'NONE',  ( -0.000000000000000000, -0.000000000000000000, 1.000000000000000000 ) ) ;
#10287=CARTESIAN_POINT ( 'NONE',  ( 30.00000000000000000, -39.99999999999999289, 52.00000000000000000 ) ) ;
#10289=AXIS2_PLACEMENT_3D ( 'NONE', #17442, #9384, #15845 ) ;
#10295=ADVANCED_FACE ( 'NONE', ( #11189 ), #4826, .T. ) ;
#10297=( NAMED_UNIT ( * ) SI_UNIT ( $, .STERADIAN. ) SOLID_ANGLE_UNIT ( ) );
#10303=CARTESIAN_POINT ( 'NONE',  ( 39.99999999999999289, -122.3205080756887639, -86.97287527660684248 ) ) ;
#10304=SURFACE_STYLE_FILL_AREA ( #11994 ) ;
#10305=LINE ( 'NONE', #10625, #7465 ) ;
#10306=CARTESIAN_POINT ( 'NONE',  ( 30.00000000000000000, 4.299168419249259188, 84.99999999999997158 ) ) ;
#10308=EDGE_CURVE ( 'NONE', #4931, #19553, #19246, .T. ) ;
#10312=CARTESIAN_POINT ( 'NONE',  ( 9.482998254698369323, -19.29932845388887586, 71.54974094241292448 ) ) ;
#10313=ORIENTED_EDGE ( 'NONE', *, *, #3743, .F. ) ;
#10318=ORIENTED_EDGE ( 'NONE', *, *, #13882, .F. ) ;
#10328=CARTESIAN_POINT ( 'NONE',  ( 21.39608139526261255, -2.344611746178258294, -83.84634603192273516 ) ) ;
#10335=EDGE_LOOP ( 'NONE', ( #18981, #3276, #10760, #14169 ) ) ;
#10337=VERTEX_POINT ( 'NONE', #14584 ) ;
#10338=CARTESIAN_POINT ( 'NONE',  ( 50.00000000000000000, 4.299168419249259188, -90.00000000000001421 ) ) ;
#10340=ORIENTED_EDGE ( 'NONE', *, *, #14879, .F. ) ;
#10344=CARTESIAN_POINT ( 'NONE',  ( -30.00000000000000000, -85.00000000000000000, -9.000000000000005329 ) ) ;
#10352=PLANE ( 'NONE',  #7428 ) ;
#10356=CIRCLE ( 'NONE', #3249, 3.199999999999994404 ) ;
#10367=EDGE_CURVE ( 'NONE', #8060, #3623, #7702, .T. ) ;
#10368=VERTEX_POINT ( 'NONE', #957 ) ;
#10372=VECTOR ( 'NONE', #3050, 1000.000000000000000 ) ;
#10374=CYLINDRICAL_SURFACE ( 'NONE', #18359, 21.50000000000000000 ) ;
#10375=EDGE_CURVE ( 'NONE', #5100, #5928, #9399, .T. ) ;
#10377=CIRCLE ( 'NONE', #5285, 8.999999999999994671 ) ;
#10390=DIRECTION ( 'NONE',  ( 1.000000000000000000, 0.000000000000000000, 0.000000000000000000 ) ) ;
#10393=FACE_OUTER_BOUND ( 'NONE', #11343, .T. ) ;
#10401=EDGE_LOOP ( 'NONE', ( #10918, #8726 ) ) ;
#10402=DIRECTION ( 'NONE',  ( 0.000000000000000000, 0.000000000000000000, 1.000000000000000000 ) ) ;
#10405=DIRECTION ( 'NONE',  ( 0.000000000000000000, 0.000000000000000000, -1.000000000000000000 ) ) ;
#10410=CARTESIAN_POINT ( 'NONE',  ( 30.88344783082026979, -110.8959383681548303, -79.30904931452684536 ) ) ;
#10422=VERTEX_POINT ( 'NONE', #18272 ) ;
#10423=CARTESIAN_POINT ( 'NONE',  ( -24.99999999999999289, -160.0000000000000000, 53.99496054166690584 ) ) ;
#10432=CARTESIAN_POINT ( 'NONE',  ( -30.00000000000000000, -85.00000000000000000, 79.99999999999998579 ) ) ;
#10438=VERTEX_POINT ( 'NONE', #5125 ) ;
#10439=CARTESIAN_POINT ( 'NONE',  ( 20.23544477270225173, -7.290198706429629638, -79.18558687180571098 ) ) ;
#10440=VERTEX_POINT ( 'NONE', #5240 ) ;
#10442=DIRECTION ( 'NONE',  ( 0.000000000000000000, 0.000000000000000000, -1.000000000000000000 ) ) ;
#10446=ORIENTED_EDGE ( 'NONE', *, *, #10110, .T. ) ;
#10453=ADVANCED_FACE ( 'NONE', ( #3339 ), #8209, .T. ) ;
#10463=DIRECTION ( 'NONE',  ( -1.000000000000000000, -0.000000000000000000, -0.000000000000000000 ) ) ;
#10468=EDGE_CURVE ( 'NONE', #13280, #11798, #9658, .T. ) ;
#10469=VERTEX_POINT ( 'NONE', #586 ) ;
#10470=CARTESIAN_POINT ( 'NONE',  ( -24.99999999999999289, 31.35083268962912584, 6.892027480330899929E-14 ) ) ;
#10479=CARTESIAN_POINT ( 'NONE',  ( 50.00000000000000000, -139.6410161513775563, -82.60203400177307742 ) ) ;
#10491=DIRECTION ( 'NONE',  ( 0.000000000000000000, 0.000000000000000000, 1.000000000000000000 ) ) ;
#10499=ORIENTED_EDGE ( 'NONE', *, *, #10568, .T. ) ;
#10500=FACE_OUTER_BOUND ( 'NONE', #14878, .T. ) ;
#10501=MECHANICAL_DESIGN_GEOMETRIC_PRESENTATION_REPRESENTATION('',(#15229),#22);
#10504=ADVANCED_FACE ( 'NONE', ( #8413 ), #19646, .F. ) ;
#10508=CARTESIAN_POINT ( 'NONE',  ( 50.00000000000000000, 230.0000000000000000, -84.99999999999998579 ) ) ;
#10513=FACE_OUTER_BOUND ( 'NONE', #4066, .T. ) ;
#10517=CARTESIAN_POINT ( 'NONE',  ( 9.140901424055382307, -19.46372757881361437, 71.47335990888086599 ) ) ;
#10522=VERTEX_POINT ( 'NONE', #15410 ) ;
#10523=CARTESIAN_POINT ( 'NONE',  ( 50.00000000000000000, -1.326995226329880762, -84.99999999999998579 ) ) ;
#10540=ORIENTED_EDGE ( 'NONE', *, *, #1711, .T. ) ;
#10541=CARTESIAN_POINT ( 'NONE',  ( 2.601994274788645534, -21.34541601844983560, -70.64469287327101199 ) ) ;
#10545=CARTESIAN_POINT ( 'NONE',  ( -24.99999999999999289, -40.41646384503856382, 66.42520834682601105 ) ) ;
#10552=VERTEX_POINT ( 'NONE', #5542 ) ;
#10563=EDGE_LOOP ( 'NONE', ( #20893, #6186, #8397, #12273 ) ) ;
#10564=CARTESIAN_POINT ( 'NONE',  ( -12.58049110815190730, -17.44827660000074232, 78.15203050255141193 ) ) ;
#10566=CARTESIAN_POINT ( 'NONE',  ( -24.99999999999999289, -85.00000000000000000, -1.040949779275250179E-14 ) ) ;
#10568=EDGE_CURVE ( 'NONE', #1127, #10422, #20383, .T. ) ;
#10579=ORIENTED_EDGE ( 'NONE', *, *, #2852, .F. ) ;
#10580=CIRCLE ( 'NONE', #13292, 14.49999999999999467 ) ;
#10603=FACE_OUTER_BOUND ( 'NONE', #259, .T. ) ;
#10607=VERTEX_POINT ( 'NONE', #11267 ) ;
#10609=LINE ( 'NONE', #5401, #17490 ) ;
#10625=CARTESIAN_POINT ( 'NONE',  ( 30.00000000000000000, -85.00000000000000000, 79.99999999999998579 ) ) ;
#10628=ORIENTED_EDGE ( 'NONE', *, *, #17268, .T. ) ;
#10632=CARTESIAN_POINT ( 'NONE',  ( -6.110423144575286791, -20.66992657861277038, 70.93137971084414062 ) ) ;
#10642=DIRECTION ( 'NONE',  ( 0.000000000000000000, 0.000000000000000000, -1.000000000000000000 ) ) ;
#10654=DIRECTION ( 'NONE',  ( 0.000000000000000000, 0.000000000000000000, -1.000000000000000000 ) ) ;
#10657=CARTESIAN_POINT ( 'NONE',  ( 2.985015299703236646, -21.29524168283703744, -70.66569055735612892 ) ) ;
#10666=CIRCLE ( 'NONE', #12357, 20.00000000000000000 ) ;
#10677=PLANE ( 'NONE',  #17707 ) ;
#10679=CARTESIAN_POINT ( 'NONE',  ( -17.90548703470696879, -11.90519517575888919, 81.89175300428205162 ) ) ;
#10685=LINE ( 'NONE', #17354, #4980 ) ;
#10686=DIRECTION ( 'NONE',  ( 0.000000000000000000, 0.000000000000000000, -1.000000000000000000 ) ) ;
#10687=ORIENTED_EDGE ( 'NONE', *, *, #20764, .F. ) ;
#10688=CARTESIAN_POINT ( 'NONE',  ( 15.22879382678786975, -17.29418148938178845, -78.22818066287017302 ) ) ;
#10704=VERTEX_POINT ( 'NONE', #17635 ) ;
#10706=AXIS2_PLACEMENT_3D ( 'NONE', #112, #16226, #18019 ) ;
#10714=VERTEX_POINT ( 'NONE', #7773 ) ;
#10715=FACE_OUTER_BOUND ( 'NONE', #3858, .T. ) ;
#10717=DIRECTION ( 'NONE',  ( 1.000000000000000000, 0.000000000000000000, 0.000000000000000000 ) ) ;
#10721=ORIENTED_EDGE ( 'NONE', *, *, #631, .T. ) ;
#10734=CARTESIAN_POINT ( 'NONE',  ( 50.00000000000000000, -30.00000000000000711, 44.99999999999998579 ) ) ;
#10737=STYLED_ITEM ( 'NONE', ( #447 ), #3656 ) ;
#10738=CARTESIAN_POINT ( 'NONE',  ( 0.000000000000000000, 0.000000000000000000, -81.99999999999998579 ) ) ;
#10741=FACE_OUTER_BOUND ( 'NONE', #3887, .T. ) ;
#10752=CARTESIAN_POINT ( 'NONE',  ( 30.00000000000000000, -122.0000000000000000, 2.099999999999984102 ) ) ;
#10757=EDGE_LOOP ( 'NONE', ( #9560, #8858, #639, #687, #4667, #18304 ) ) ;
#10760=ORIENTED_EDGE ( 'NONE', *, *, #9606, .T. ) ;
#10762=FACE_OUTER_BOUND ( 'NONE', #18215, .T. ) ;
#10775=CARTESIAN_POINT ( 'NONE',  ( 31.94921915542539637, -113.6563480467028029, 75.04517990444932707 ) ) ;
#10776=DIRECTION ( 'NONE',  ( 1.000000000000000000, 0.000000000000000000, 0.000000000000000000 ) ) ;
#10778=VERTEX_POINT ( 'NONE', #10752 ) ;
#10781=CARTESIAN_POINT ( 'NONE',  ( -18.38761746031185496, -11.14595575959862295, 82.49318946023234389 ) ) ;
#10793=CARTESIAN_POINT ( 'NONE',  ( 4.250247840617388917, -22.60715243308596101, -75.54244079978928994 ) ) ;
#10798=FACE_OUTER_BOUND ( 'NONE', #17338, .T. ) ;
#10800=DIRECTION ( 'NONE',  ( -1.000000000000000000, 0.000000000000000000, 0.000000000000000000 ) ) ;
#10806=ORIENTED_EDGE ( 'NONE', *, *, #3284, .F. ) ;
#10815=ORIENTED_EDGE ( 'NONE', *, *, #410, .T. ) ;
#10818=DIRECTION ( 'NONE',  ( 0.000000000000000000, 0.000000000000000000, -1.000000000000000000 ) ) ;
#10819=CARTESIAN_POINT ( 'NONE',  ( 30.00000000000000000, -39.99999999999999289, -54.09999999999999432 ) ) ;
#10824=DIRECTION ( 'NONE',  ( 0.000000000000000000, -0.000000000000000000, 1.000000000000000000 ) ) ;
#10826=DIRECTION ( 'NONE',  ( 1.000000000000000000, 0.000000000000000000, 0.000000000000000000 ) ) ;
#10828=DIRECTION ( 'NONE',  ( 1.000000000000000000, 0.000000000000000000, 0.000000000000000000 ) ) ;
#10831=CARTESIAN_POINT ( 'NONE',  ( 0.000000000000000000, 0.000000000000000000, -81.99999999999998579 ) ) ;
#10832=VERTEX_POINT ( 'NONE', #11158 ) ;
#10834=CARTESIAN_POINT ( 'NONE',  ( 21.45900938229203447, -1.326995226329893862, 84.99999999999998579 ) ) ;
#10837=ORIENTED_EDGE ( 'NONE', *, *, #11038, .T. ) ;
#10859=DIRECTION ( 'NONE',  ( 0.000000000000000000, 0.000000000000000000, -1.000000000000000000 ) ) ;
#10886=CARTESIAN_POINT ( 'NONE',  ( 21.29589421403332494, -8.772909163211549455, -84.50987075322080955 ) ) ;
#10890=ORIENTED_EDGE ( 'NONE', *, *, #1838, .F. ) ;
#10893=DIRECTION ( 'NONE',  ( 1.000000000000000000, -0.000000000000000000, -0.000000000000000000 ) ) ;
#10905=AXIS2_PLACEMENT_3D ( 'NONE', #16524, #16037, #13459 ) ;
#10909=CARTESIAN_POINT ( 'NONE',  ( 30.00000000000000000, -105.0000000000000000, 72.35596062816881613 ) ) ;
#10911=ORIENTED_EDGE ( 'NONE', *, *, #668, .T. ) ;
#10912=EDGE_CURVE ( 'NONE', #19648, #17002, #9687, .T. ) ;
#10915=CARTESIAN_POINT ( 'NONE',  ( 37.45104809098000942, -20.09218443038071200, -76.71572404264729528 ) ) ;
#10916=DIRECTION ( 'NONE',  ( 0.000000000000000000, 0.000000000000000000, 1.000000000000000000 ) ) ;
#10918=ORIENTED_EDGE ( 'NONE', *, *, #19061, .T. ) ;
#10919=CARTESIAN_POINT ( 'NONE',  ( 34.73553668442697528, -117.9508568039212832, -77.26256316625480736 ) ) ;
#10925=EDGE_CURVE ( 'NONE', #15704, #15337, #17131, .T. ) ;
#10932=DIRECTION ( 'NONE',  ( 1.000000000000000000, 0.000000000000000000, 0.000000000000000000 ) ) ;
#10933=ORIENTED_EDGE ( 'NONE', *, *, #20220, .F. ) ;
#10934=CARTESIAN_POINT ( 'NONE',  ( 30.00000000000000000, -85.00000000000000000, -1.040949779275250179E-14 ) ) ;
#10937=CARTESIAN_POINT ( 'NONE',  ( 15.37884418493264782, -15.02891098528242431, 73.77646566961476537 ) ) ;
#10940=EDGE_CURVE ( 'NONE', #8249, #7867, #20254, .T. ) ;
#10947=CARTESIAN_POINT ( 'NONE',  ( -44.00000000000000000, -85.00000000000000000, 11.49999999999998579 ) ) ;
#10952=CIRCLE ( 'NONE', #2495, 80.00000000000000000 ) ;
#10963=ORIENTED_EDGE ( 'NONE', *, *, #19234, .T. ) ;
#10973=AXIS2_PLACEMENT_3D ( 'NONE', #12101, #449, #11781 ) ;
#10977=CIRCLE ( 'NONE', #11651, 39.99999999999999289 ) ;
#10979=ORIENTED_EDGE ( 'NONE', *, *, #12855, .T. ) ;
#10981=EDGE_CURVE ( 'NONE', #4783, #13795, #3900, .T. ) ;
#10984=CARTESIAN_POINT ( 'NONE',  ( 20.20955665649389843, -7.405347705393168667, 85.81428755717244883 ) ) ;
#10988=ORIENTED_EDGE ( 'NONE', *, *, #20220, .T. ) ;
#10991=ORIENTED_EDGE ( 'NONE', *, *, #12420, .F. ) ;
#10992=CARTESIAN_POINT ( 'NONE',  ( -21.27651084028035910, -8.819135707481013497, -84.46788585316646447 ) ) ;
#10995=VERTEX_POINT ( 'NONE', #7855 ) ;
#11009=EDGE_CURVE ( 'NONE', #8953, #8874, #17410, .T. ) ;
#11020=CARTESIAN_POINT ( 'NONE',  ( 30.89068055997971385, -39.25147108719813360, -71.46578918091849175 ) ) ;
#11021=LINE ( 'NONE', #10819, #19730 ) ;
#11026=AXIS2_PLACEMENT_3D ( 'NONE', #1769, #11313, #9917 ) ;
#11027=B_SPLINE_CURVE_WITH_KNOTS ( 'NONE', 3,
 ( #916, #12566, #12363, #13844, #9284, #12469, #4303, #10775, #15633, #7584, #20512, #15745, #1242, #14172, #1659, #1554, #8306, #6503, #4923, #9795 ),
 .UNSPECIFIED., .F., .F.,
 ( 4, 2, 2, 2, 2, 2, 2, 2, 2, 4 ),
 ( 0.000000000000000000, 0.005578321817708520487, 0.006972902272135647790, 0.008367482726562769021, 0.01115664363541698026, 0.01255122408984410062, 0.01394580454427121752, 0.01673496545312545478, 0.01952412636197969203, 0.02231328727083392929 ),
 .UNSPECIFIED. ) ;
#11029=PLANE ( 'NONE',  #15004 ) ;
#11038=EDGE_CURVE ( 'NONE', #13702, #2306, #17821, .T. ) ;
#11040=ORIENTED_EDGE ( 'NONE', *, *, #14301, .T. ) ;
#11046=CARTESIAN_POINT ( 'NONE',  ( 50.00000000000000000, -42.57363661491096707, -121.3828884801879155 ) ) ;
#11052=CARTESIAN_POINT ( 'NONE',  ( -25.00000000000000000, -30.00000000000000711, 50.99019513592783426 ) ) ;
#11053=DIRECTION ( 'NONE',  ( 0.000000000000000000, -1.000000000000000000, -0.000000000000000000 ) ) ;
#11055=ADVANCED_FACE ( 'NONE', ( #18785 ), #4254, .T. ) ;
#11061=VECTOR ( 'NONE', #16988, 1000.000000000000000 ) ;
#11062=CIRCLE ( 'NONE', #4626, 23.00000000000000000 ) ;
#11077=ADVANCED_FACE ( 'NONE', ( #3083 ), #7967, .T. ) ;
#11084=DIRECTION ( 'NONE',  ( -0.000000000000000000, -1.000000000000000000, -0.000000000000000000 ) ) ;
#11085=AXIS2_PLACEMENT_3D ( 'NONE', #12385, #7722, #15549 ) ;
#11089=DIRECTION ( 'NONE',  ( 1.000000000000000000, -0.000000000000000000, -0.000000000000000000 ) ) ;
#11094=AXIS2_PLACEMENT_3D ( 'NONE', #17871, #11089, #7896 ) ;
#11098=AXIS2_PLACEMENT_3D ( 'NONE', #8134, #7824, #20549 ) ;
#11108=LINE ( 'NONE', #14703, #11620 ) ;
#11111=ORIENTED_EDGE ( 'NONE', *, *, #14047, .F. ) ;
#11120=DIRECTION ( 'NONE',  ( 0.000000000000000000, 0.000000000000000000, 1.000000000000000000 ) ) ;
#11122=DIRECTION ( 'NONE',  ( 1.000000000000000000, -0.000000000000000000, -0.000000000000000000 ) ) ;
#11128=CARTESIAN_POINT ( 'NONE',  ( 31.38212025810754824, -36.77472472338947540, -71.71337048941178693 ) ) ;
#11130=EDGE_CURVE ( 'NONE', #3436, #8121, #11545, .T. ) ;
#11132=ORIENTED_EDGE ( 'NONE', *, *, #5387, .T. ) ;
#11133=LINE ( 'NONE', #3072, #14122 ) ;
#11140=CARTESIAN_POINT ( 'NONE',  ( -44.00000000000000000, -85.00000000000000000, -1.040949779275250179E-14 ) ) ;
#11143=EDGE_CURVE ( 'NONE', #2306, #13702, #16439, .T. ) ;
#11148=DIRECTION ( 'NONE',  ( 1.000000000000000000, 0.000000000000000000, 0.000000000000000000 ) ) ;
#11150=CARTESIAN_POINT ( 'NONE',  ( -8.500000000000000000, 0.000000000000000000, -81.99999999999998579 ) ) ;
#11154=CARTESIAN_POINT ( 'NONE',  ( 30.00000000000000000, -85.00000000000000000, -1.040949779275250179E-14 ) ) ;
#11158=CARTESIAN_POINT ( 'NONE',  ( 25.00000000000000711, -29.99999999999999645, -45.00000000000000000 ) ) ;
#11162=DIRECTION ( 'NONE',  ( -1.000000000000000000, 0.000000000000000000, 0.000000000000000000 ) ) ;
#11165=EDGE_CURVE ( 'NONE', #14747, #14238, #3387, .T. ) ;
#11175=ORIENTED_EDGE ( 'NONE', *, *, #18305, .F. ) ;
#11176=DIRECTION ( 'NONE',  ( -0.000000000000000000, -0.000000000000000000, 1.000000000000000000 ) ) ;
#11178=LINE ( 'NONE', #15943, #13271 ) ;
#11180=ORIENTED_EDGE ( 'NONE', *, *, #15687, .F. ) ;
#11181=ADVANCED_FACE ( 'NONE', ( #16018 ), #13155, .F. ) ;
#11189=FACE_OUTER_BOUND ( 'NONE', #16058, .T. ) ;
#11191=DIRECTION ( 'NONE',  ( -1.000000000000000000, 0.000000000000000000, 0.000000000000000000 ) ) ;
#11195=DIRECTION ( 'NONE',  ( 0.000000000000000000, 0.000000000000000000, -1.000000000000000000 ) ) ;
#11200=CARTESIAN_POINT ( 'NONE',  ( 0.000000000000000000, 0.000000000000000000, 68.00000000000000000 ) ) ;
#11201=CIRCLE ( 'NONE', #35, 11.49999999999999645 ) ;
#11203=CARTESIAN_POINT ( 'NONE',  ( -20.20451054323269346, -11.00838379098076025, -82.59978733170636644 ) ) ;
#11214=AXIS2_PLACEMENT_3D ( 'NONE', #4668, #18880, #10818 ) ;
#11220=EDGE_LOOP ( 'NONE', ( #20195, #17119 ) ) ;
#11222=CYLINDRICAL_SURFACE ( 'NONE', #18171, 80.00000000000000000 ) ;
#11223=CARTESIAN_POINT ( 'NONE',  ( 30.00000000000000000, -50.00000000000000000, 66.88656633939929463 ) ) ;
#11226=DIRECTION ( 'NONE',  ( 1.000000000000000000, 0.000000000000000000, 0.000000000000000000 ) ) ;
#11227=VECTOR ( 'NONE', #13643, 1000.000000000000000 ) ;
#11232=CIRCLE ( 'NONE', #2086, 5.000000000000004441 ) ;
#11233=ORIENTED_EDGE ( 'NONE', *, *, #18305, .T. ) ;
#11235=CARTESIAN_POINT ( 'NONE',  ( 0.000000000000000000, 0.000000000000000000, -130.0000000000000000 ) ) ;
#11241=DIRECTION ( 'NONE',  ( 0.000000000000000000, 0.000000000000000000, -1.000000000000000000 ) ) ;
#11243=DIRECTION ( 'NONE',  ( 0.000000000000000000, 0.000000000000000000, 1.000000000000000000 ) ) ;
#11254=CARTESIAN_POINT ( 'NONE',  ( 32.75992285807288340, -31.42540396991885032, 72.63203971126306158 ) ) ;
#11257=LINE ( 'NONE', #7660, #9332 ) ;
#11260=AXIS2_PLACEMENT_3D ( 'NONE', #3567, #84, #6845 ) ;
#11263=DIRECTION ( 'NONE',  ( 0.000000000000000000, 1.040834085586084454E-15, -1.000000000000000000 ) ) ;
#11267=CARTESIAN_POINT ( 'NONE',  ( 21.50000000000000000, 0.000000000000000000, 68.00000000000000000 ) ) ;
#11269=AXIS2_PLACEMENT_3D ( 'NONE', #14707, #19571, #17984 ) ;
#11270=CARTESIAN_POINT ( 'NONE',  ( 24.99999999999999289, -30.00000000000000711, 44.99999999999998579 ) ) ;
#11272=VECTOR ( 'NONE', #17995, 1000.000000000000000 ) ;
#11277=CARTESIAN_POINT ( 'NONE',  ( 40.00000000000000711, -40.00000000000001421, -130.0000000000000000 ) ) ;
#11278=ORIENTED_EDGE ( 'NONE', *, *, #13304, .T. ) ;
#11290=CARTESIAN_POINT ( 'NONE',  ( 50.00000000000000000, -124.9999999999999858, 90.00000000000001421 ) ) ;
#11295=ORIENTED_EDGE ( 'NONE', *, *, #18534, .F. ) ;
#11298=CIRCLE ( 'NONE', #129, 80.00000000000000000 ) ;
#11299=EDGE_CURVE ( 'NONE', #3180, #10778, #19479, .T. ) ;
#11308=EDGE_CURVE ( 'NONE', #17074, #14667, #6628, .T. ) ;
#11309=DIRECTION ( 'NONE',  ( 0.000000000000000000, -1.000000000000000000, -8.673617379884036705E-17 ) ) ;
#11313=DIRECTION ( 'NONE',  ( -1.000000000000000000, 0.000000000000000000, 0.000000000000000000 ) ) ;
#11316=AXIS2_PLACEMENT_3D ( 'NONE', #3406, #11471, #17846 ) ;
#11317=ORIENTED_EDGE ( 'NONE', *, *, #17139, .T. ) ;
#11328=EDGE_CURVE ( 'NONE', #8874, #4685, #7481, .T. ) ;
#11330=FACE_OUTER_BOUND ( 'NONE', #10563, .T. ) ;
#11331=VERTEX_POINT ( 'NONE', #14844 ) ;
#11337=LINE ( 'NONE', #11441, #4482 ) ;
#11340=FACE_BOUND ( 'NONE', #20596, .T. ) ;
#11341=DIRECTION ( 'NONE',  ( -1.000000000000000000, 0.000000000000000000, 0.000000000000000000 ) ) ;
#11343=EDGE_LOOP ( 'NONE', ( #19545, #17433, #15249, #9137, #2900, #6059, #14484, #4564 ) ) ;
#11355=CARTESIAN_POINT ( 'NONE',  ( 30.00000000000000000, -30.00000000000000711, 58.09475019311124555 ) ) ;
#11356=ORIENTED_EDGE ( 'NONE', *, *, #3012, .F. ) ;
#11357=CYLINDRICAL_SURFACE ( 'NONE', #8530, 8.500000000000000000 ) ;
#11359=CARTESIAN_POINT ( 'NONE',  ( 50.00000000000000000, -124.9999999999999858, -90.00000000000001421 ) ) ;
#11361=CYLINDRICAL_SURFACE ( 'NONE', #7214, 20.00000000000000355 ) ;
#11362=ORIENTED_EDGE ( 'NONE', *, *, #4439, .T. ) ;
#11367=ORIENTED_EDGE ( 'NONE', *, *, #17015, .T. ) ;
#11369=EDGE_CURVE ( 'NONE', #5841, #18257, #16629, .T. ) ;
#11373=DIRECTION ( 'NONE',  ( 1.000000000000000000, 0.000000000000000000, 0.000000000000000000 ) ) ;
#11374=ORIENTED_EDGE ( 'NONE', *, *, #15850, .F. ) ;
#11383=CYLINDRICAL_SURFACE ( 'NONE', #2754, 20.00000000000000355 ) ;
#11385=LINE ( 'NONE', #19538, #16712 ) ;
#11400=ORIENTED_EDGE ( 'NONE', *, *, #20764, .T. ) ;
#11401=CARTESIAN_POINT ( 'NONE',  ( -20.48001470518130773, -6.654962914332837265, -79.70582905289667508 ) ) ;
#11404=CARTESIAN_POINT ( 'NONE',  ( -30.00000000000000000, 36.35083268962917202, 90.00000000000000000 ) ) ;
#11411=CARTESIAN_POINT ( 'NONE',  ( 30.00000000000000711, -40.00000000000001421, -130.0000000000000000 ) ) ;
#11412=ORIENTED_EDGE ( 'NONE', *, *, #13253, .F. ) ;
#11413=FACE_OUTER_BOUND ( 'NONE', #19039, .T. ) ;
#11415=DIRECTION ( 'NONE',  ( -0.6156453966108028641, 0.000000000000000000, -0.7880233154113698291 ) ) ;
#11416=B_SPLINE_CURVE_WITH_KNOTS ( 'NONE', 3,
 ( #17907, #3367, #9832, #8141, #19377, #20862, #12831, #9742, #13139, #19586, #1789, #8245, #11523, #17997, #4756, #9936, #8350, #1694, #14828, #12726, #4663, #11223 ),
 .UNSPECIFIED., .F., .F.,
 ( 4, 2, 2, 2, 2, 2, 2, 2, 2, 2, 4 ),
 ( 0.008203449124722041533, 0.01993989471859326790, 0.02287400611706106451, 0.02580811751552886807, 0.03167634031246444049, 0.03461045171093222322, 0.03754456310939999902, 0.04341278590633557144, 0.04928100870327114386, 0.05221512010173892659, 0.05514923150020671627 ),
 .UNSPECIFIED. ) ;
#11418=ORIENTED_EDGE ( 'NONE', *, *, #7392, .T. ) ;
#11419=CARTESIAN_POINT ( 'NONE',  ( 30.00000000000000000, -170.8299878242309546, -15.48896927112552824 ) ) ;
#11421=DIRECTION ( 'NONE',  ( 1.000000000000000000, 0.000000000000000000, 0.000000000000000000 ) ) ;
#11430=FACE_BOUND ( 'NONE', #5977, .T. ) ;
#11432=DIRECTION ( 'NONE',  ( -0.000000000000000000, -1.000000000000000000, -0.000000000000000000 ) ) ;
#11435=ORIENTED_EDGE ( 'NONE', *, *, #14701, .F. ) ;
#11439=DIRECTION ( 'NONE',  ( 0.000000000000000000, -1.000000000000000000, 0.000000000000000000 ) ) ;
#11441=CARTESIAN_POINT ( 'NONE',  ( 50.00000000000000000, 230.0000000000000000, 84.99999999999998579 ) ) ;
#11445=DIRECTION ( 'NONE',  ( 0.000000000000000000, 0.000000000000000000, -1.000000000000000000 ) ) ;
#11446=ORIENTED_EDGE ( 'NONE', *, *, #17982, .T. ) ;
#11447=EDGE_CURVE ( 'NONE', #4931, #18682, #17669, .T. ) ;
#11457=DIRECTION ( 'NONE',  ( 1.000000000000000000, 0.000000000000000000, 0.000000000000000000 ) ) ;
#11467=CARTESIAN_POINT ( 'NONE',  ( 33.23318211478949991, -29.69549557693871833, -67.81563648932102240 ) ) ;
#11471=DIRECTION ( 'NONE',  ( 1.000000000000000000, -0.000000000000000000, -0.000000000000000000 ) ) ;
#11478=EDGE_LOOP ( 'NONE', ( #4977, #1961 ) ) ;
#11492=ORIENTED_EDGE ( 'NONE', *, *, #14253, .F. ) ;
#11498=CARTESIAN_POINT ( 'NONE',  ( 30.00000000000000355, -139.6410161513775563, -90.00000000000001421 ) ) ;
#11500=DIRECTION ( 'NONE',  ( -1.000000000000000000, 0.000000000000000000, 0.000000000000000000 ) ) ;
#11507=COLOUR_RGB ( '', 0.66274510, 0.83137255, 0.94901961) ;
#11508=ORIENTED_EDGE ( 'NONE', *, *, #10249, .F. ) ;
#11513=VERTEX_POINT ( 'NONE', #2936 ) ;
#11518=PLANE ( 'NONE',  #4827 ) ;
#11523=CARTESIAN_POINT ( 'NONE',  ( 32.70638587058282098, -31.60219482138385061, 67.47980676442061565 ) ) ;
#11528=LINE ( 'NONE', #11844, #15291 ) ;
#11529=CARTESIAN_POINT ( 'NONE',  ( 50.00000000000000000, 230.0000000000000000, 0.000000000000000000 ) ) ;
#11531=AXIS2_PLACEMENT_3D ( 'NONE', #2275, #12020, #15201 ) ;
#11533=ORIENTED_EDGE ( 'NONE', *, *, #548, .T. ) ;
#11534=CARTESIAN_POINT ( 'NONE',  ( 45.73369142091321748, -8.073147882754625471, 78.54250490773422655 ) ) ;
#11545=LINE ( 'NONE', #6674, #2909 ) ;
#11554=VERTEX_POINT ( 'NONE', #20526 ) ;
#11559=CARTESIAN_POINT ( 'NONE',  ( 30.75237355671447048, -40.04063416367457506, 71.40923356276123002 ) ) ;
#11573=CARTESIAN_POINT ( 'NONE',  ( 31.02182833614992674, -111.3267134195865395, -79.49107265470053107 ) ) ;
#11575=CARTESIAN_POINT ( 'NONE',  ( 30.00000000000000000, -99.99999999999998579, 52.00000000000000000 ) ) ;
#11578=ORIENTED_EDGE ( 'NONE', *, *, #4679, .T. ) ;
#11589=FACE_OUTER_BOUND ( 'NONE', #13225, .T. ) ;
#11593=DIRECTION ( 'NONE',  ( 1.000000000000000000, -0.000000000000000000, -0.000000000000000000 ) ) ;
#11601=AXIS2_PLACEMENT_3D ( 'NONE', #8673, #16527, #13356 ) ;
#11605=ORIENTED_EDGE ( 'NONE', *, *, #11908, .F. ) ;
#11612=ORIENTED_EDGE ( 'NONE', *, *, #14429, .T. ) ;
#11615=ORIENTED_EDGE ( 'NONE', *, *, #7252, .F. ) ;
#11620=VECTOR ( 'NONE', #11415, 1000.000000000000000 ) ;
#11639=CARTESIAN_POINT ( 'NONE',  ( 30.00000000000000355, -139.6410161513775563, -85.00000000000000000 ) ) ;
#11640=ORIENTED_EDGE ( 'NONE', *, *, #18263, .T. ) ;
#11645=CARTESIAN_POINT ( 'NONE',  ( 24.99999999999999645, -85.00000000000000000, 75.00000000000000000 ) ) ;
#11648=CARTESIAN_POINT ( 'NONE',  ( 21.50000000000000000, 0.000000000000000000, 84.99999999999998579 ) ) ;
#11651=AXIS2_PLACEMENT_3D ( 'NONE', #11899, #10212, #20160 ) ;
#11661=DIRECTION ( 'NONE',  ( 0.000000000000000000, 0.000000000000000000, 1.000000000000000000 ) ) ;
#11668=ORIENTED_EDGE ( 'NONE', *, *, #8747, .F. ) ;
#11679=CARTESIAN_POINT ( 'NONE',  ( 38.54445100392999990, -121.4157858342328495, -86.08560793638669395 ) ) ;
#11687=ADVANCED_FACE ( 'NONE', ( #19874 ), #8422, .T. ) ;
#11690=ORIENTED_EDGE ( 'NONE', *, *, #1838, .T. ) ;
#11691=LINE ( 'NONE', #16560, #14008 ) ;
#11705=CARTESIAN_POINT ( 'NONE',  ( 30.00000000000000000, -170.8299878242309546, 15.48896927112552824 ) ) ;
#11710=ADVANCED_FACE ( 'NONE', ( #1764 ), #8217, .T. ) ;
#11711=DIRECTION ( 'NONE',  ( 0.000000000000000000, 0.000000000000000000, 1.000000000000000000 ) ) ;
#11712=ORIENTED_EDGE ( 'NONE', *, *, #10981, .F. ) ;
#11714=ORIENTED_EDGE ( 'NONE', *, *, #2472, .T. ) ;
#11717=CARTESIAN_POINT ( 'NONE',  ( 50.00000000000000000, -170.8299878242309546, 15.48896927112552824 ) ) ;
#11718=VERTEX_POINT ( 'NONE', #3443 ) ;
#11725=ORIENTED_EDGE ( 'NONE', *, *, #17772, .F. ) ;
#11727=VECTOR ( 'NONE', #8723, 1000.000000000000000 ) ;
#11740=VERTEX_POINT ( 'NONE', #19963 ) ;
#11744=VERTEX_POINT ( 'NONE', #13619 ) ;
#11747=CARTESIAN_POINT ( 'NONE',  ( 30.00000000000000000, -164.9999999999999716, 50.00000000000001421 ) ) ;
#11761=VECTOR ( 'NONE', #3043, 1000.000000000000000 ) ;
#11764=DIRECTION ( 'NONE',  ( 0.000000000000000000, -1.000000000000000000, 0.000000000000000000 ) ) ;
#11770=LINE ( 'NONE', #7085, #17080 ) ;
#11773=VERTEX_POINT ( 'NONE', #10545 ) ;
#11774=FACE_BOUND ( 'NONE', #19439, .T. ) ;
#11779=ADVANCED_FACE ( 'NONE', ( #20396, #20068 ), #20281, .F. ) ;
#11781=DIRECTION ( 'NONE',  ( -1.000000000000000000, 0.000000000000000000, 0.000000000000000000 ) ) ;
#11782=EDGE_CURVE ( 'NONE', #14994, #17908, #2604, .T. ) ;
#11792=CARTESIAN_POINT ( 'NONE',  ( -7.539743116613911944, -20.19060691129837437, 71.13878616268864619 ) ) ;
#11796=LINE ( 'NONE', #5229, #12890 ) ;
#11798=VERTEX_POINT ( 'NONE', #3963 ) ;
#11801=DIRECTION ( 'NONE',  ( 1.000000000000000000, -0.000000000000000000, -0.000000000000000000 ) ) ;
#11806=ADVANCED_FACE ( 'NONE', ( #7042 ), #7135, .F. ) ;
#11811=ORIENTED_EDGE ( 'NONE', *, *, #15288, .F. ) ;
#11812=CARTESIAN_POINT ( 'NONE',  ( -19.56401537842534921, -8.921674172384493673, -77.87798366923529159 ) ) ;
#11819=EDGE_LOOP ( 'NONE', ( #5552, #4308 ) ) ;
#11822=CARTESIAN_POINT ( 'NONE',  ( 30.00000000000000000, -159.9999999999999716, -53.99496054166690584 ) ) ;
#11823=EDGE_CURVE ( 'NONE', #10704, #12901, #5550, .T. ) ;
#11825=ORIENTED_EDGE ( 'NONE', *, *, #2561, .F. ) ;
#11826=LINE ( 'NONE', #12142, #9050 ) ;
#11839=CARTESIAN_POINT ( 'NONE',  ( 38.20577202892028623, -121.1578191933347739, 85.85343169282300835 ) ) ;
#11841=ORIENTED_EDGE ( 'NONE', *, *, #10940, .F. ) ;
#11844=CARTESIAN_POINT ( 'NONE',  ( 50.00000000000000000, -3.649167310370820871, 90.00000000000000000 ) ) ;
#11848=DIRECTION ( 'NONE',  ( -0.000000000000000000, 1.000000000000000000, 0.000000000000000000 ) ) ;
#11849=VECTOR ( 'NONE', #7008, 1000.000000000000000 ) ;
#11854=LINE ( 'NONE', #15243, #4232 ) ;
#11858=CARTESIAN_POINT ( 'NONE',  ( 21.50000000000000000, 2.632990618166809235E-15, -68.00000000000000000 ) ) ;
#11862=AXIS2_PLACEMENT_3D ( 'NONE', #13199, #14789, #269 ) ;
#11865=ORIENTED_EDGE ( 'NONE', *, *, #4791, .F. ) ;
#11866=CARTESIAN_POINT ( 'NONE',  ( -30.00000000000000000, -170.8299878242309546, -15.48896927112552824 ) ) ;
#11869=FACE_BOUND ( 'NONE', #15872, .T. ) ;
#11874=FILL_AREA_STYLE_COLOUR ( '', #13442 ) ;
#11875=DIRECTION ( 'NONE',  ( 0.000000000000000000, -1.000000000000000000, 0.000000000000000000 ) ) ;
#11880=CARTESIAN_POINT ( 'NONE',  ( 50.00000000000000000, -3.649167310370820871, 90.00000000000000000 ) ) ;
#11885=DIRECTION ( 'NONE',  ( 0.6156453966108041964, 0.000000000000000000, -0.7880233154113687188 ) ) ;
#11893=CARTESIAN_POINT ( 'NONE',  ( 30.00000000000000711, 29.99999999999998579, -120.0000000000000142 ) ) ;
#11894=CYLINDRICAL_SURFACE ( 'NONE', #6978, 20.00000000000000355 ) ;
#11899=CARTESIAN_POINT ( 'NONE',  ( 30.00000000000000000, -97.49621075554985339, 111.6458212409894486 ) ) ;
#11903=ORIENTED_EDGE ( 'NONE', *, *, #17248, .T. ) ;
#11907=CARTESIAN_POINT ( 'NONE',  ( -18.69829135368511430, -10.63264222386860958, -76.60301815488040234 ) ) ;
#11908=EDGE_CURVE ( 'NONE', #13280, #3180, #18926, .T. ) ;
#11910=ORIENTED_EDGE ( 'NONE', *, *, #824, .T. ) ;
#11911=ADVANCED_FACE ( 'NONE', ( #1338 ), #1546, .F. ) ;
#11916=ORIENTED_EDGE ( 'NONE', *, *, #9510, .T. ) ;
#11917=ORIENTED_EDGE ( 'NONE', *, *, #17291, .F. ) ;
#11922=ORIENTED_EDGE ( 'NONE', *, *, #20111, .T. ) ;
#11927=CIRCLE ( 'NONE', #9233, 11.50000000000000000 ) ;
#11935=CARTESIAN_POINT ( 'NONE',  ( 0.000000000000000000, 0.000000000000000000, 90.00000000000000000 ) ) ;
#11939=DIRECTION ( 'NONE',  ( 1.000000000000000000, 0.000000000000000000, 0.000000000000000000 ) ) ;
#11941=VECTOR ( 'NONE', #17306, 1000.000000000000000 ) ;
#11943=EDGE_CURVE ( 'NONE', #7282, #14001, #18772, .T. ) ;
#11944=DIRECTION ( 'NONE',  ( 0.000000000000000000, 0.000000000000000000, 1.000000000000000000 ) ) ;
#11955=CIRCLE ( 'NONE', #6210, 5.000000000000004441 ) ;
#11969=CIRCLE ( 'NONE', #5182, 20.00000000000000355 ) ;
#11976=VECTOR ( 'NONE', #4700, 1000.000000000000000 ) ;
#11984=ORIENTED_EDGE ( 'NONE', *, *, #9696, .T. ) ;
#11990=AXIS2_PLACEMENT_3D ( 'NONE', #11575, #6488, #3515 ) ;
#11994=FILL_AREA_STYLE ('',( #16762 ) ) ;
#11997=ORIENTED_EDGE ( 'NONE', *, *, #6105, .F. ) ;
#12001=DIRECTION ( 'NONE',  ( 0.000000000000000000, 0.000000000000000000, -1.000000000000000000 ) ) ;
#12003=EDGE_CURVE ( 'NONE', #17173, #17850, #20441, .T. ) ;
#12009=ORIENTED_EDGE ( 'NONE', *, *, #9254, .F. ) ;
#12010=DIRECTION ( 'NONE',  ( 0.000000000000000000, 0.000000000000000000, -1.000000000000000000 ) ) ;
#12018=EDGE_LOOP ( 'NONE', ( #10120, #11984, #17958, #4473 ) ) ;
#12020=DIRECTION ( 'NONE',  ( 0.000000000000000000, 0.000000000000000000, -1.000000000000000000 ) ) ;
#12022=CARTESIAN_POINT ( 'NONE',  ( 20.90734068544160351, -5.044436930659516705, -81.16927884214386779 ) ) ;
#12028=ORIENTED_EDGE ( 'NONE', *, *, #7435, .T. ) ;
#12031=DIRECTION ( 'NONE',  ( 0.000000000000000000, 0.000000000000000000, -1.000000000000000000 ) ) ;
#12033=CARTESIAN_POINT ( 'NONE',  ( -30.00000000000000000, -85.00000000000000000, -1.040949779275250179E-14 ) ) ;
#12041=PRODUCT_CONTEXT ( 'NONE', #7078, 'mechanical' ) ;
#12047=CARTESIAN_POINT ( 'NONE',  ( -21.03332064508573396, -4.547583584323819039, 88.88568648802799999 ) ) ;
#12050=CIRCLE ( 'NONE', #4276, 2.099999999999990763 ) ;
#12058=CARTESIAN_POINT ( 'NONE',  ( -3.788816106695048536, -22.69873778718781310, -75.50243859632158205 ) ) ;
#12060=CARTESIAN_POINT ( 'NONE',  ( 45.22159793441012710, -8.673994507468391291, -90.00000000000001421 ) ) ;
#12063=EDGE_LOOP ( 'NONE', ( #14280, #2300 ) ) ;
#12069=FACE_BOUND ( 'NONE', #9172, .T. ) ;
#12075=EDGE_CURVE ( 'NONE', #11798, #13280, #15703, .T. ) ;
#12087=ORIENTED_EDGE ( 'NONE', *, *, #14193, .T. ) ;
#12088=EDGE_CURVE ( 'NONE', #2608, #19852, #11385, .T. ) ;
#12089=DIRECTION ( 'NONE',  ( 0.000000000000000000, 0.000000000000000000, 1.000000000000000000 ) ) ;
#12092=DIRECTION ( 'NONE',  ( 1.000000000000000000, 0.000000000000000000, 0.000000000000000000 ) ) ;
#12097=DIRECTION ( 'NONE',  ( 0.000000000000000000, 0.000000000000000000, -1.000000000000000000 ) ) ;
#12098=EDGE_CURVE ( 'NONE', #8802, #10552, #7934, .T. ) ;
#12101=CARTESIAN_POINT ( 'NONE',  ( -27.96694501150314593, -24.74873734152930993, -120.0000000000000142 ) ) ;
#12109=CARTESIAN_POINT ( 'NONE',  ( 30.00000000000000000, -97.49621075554985339, -111.6458212409894486 ) ) ;
#12112=CARTESIAN_POINT ( 'NONE',  ( -19.56401537842534921, -8.921674172384486567, 77.87798366923532001 ) ) ;
#12116=CARTESIAN_POINT ( 'NONE',  ( 45.41022184210711998, -126.8797397267199045, 84.49691278257978411 ) ) ;
#12118=CIRCLE ( 'NONE', #14463, 5.000000000000004441 ) ;
#12119=ORIENTED_EDGE ( 'NONE', *, *, #11823, .F. ) ;
#12131=CARTESIAN_POINT ( 'NONE',  ( -19.81419003091921383, -8.351337688303459572, -78.32518794914258820 ) ) ;
#12138=ORIENTED_EDGE ( 'NONE', *, *, #20111, .F. ) ;
#12140=EDGE_LOOP ( 'NONE', ( #12682, #2832 ) ) ;
#12142=CARTESIAN_POINT ( 'NONE',  ( 50.00000000000000000, -164.9999999999999716, -50.00000000000000711 ) ) ;
#12143=DIRECTION ( 'NONE',  ( 0.000000000000000000, 0.000000000000000000, -1.000000000000000000 ) ) ;
#12150=CARTESIAN_POINT ( 'NONE',  ( -16.04895590985772458, -14.36624353526105402, 80.08463211907583457 ) ) ;
#12155=CARTESIAN_POINT ( 'NONE',  ( 31.47548550611441343, -112.5521019397693436, 80.04644125633257090 ) ) ;
#12158=CARTESIAN_POINT ( 'NONE',  ( 2.723238954207318319, -22.84144205494821023, -75.44116118571403717 ) ) ;
#12159=VERTEX_POINT ( 'NONE', #3420 ) ;
#12164=CARTESIAN_POINT ( 'NONE',  ( 47.57345354676051130, -5.300163754693015150, -88.03325769612199281 ) ) ;
#12167=CARTESIAN_POINT ( 'NONE',  ( 8.500000000000000000, 1.040949779275250140E-15, -81.99999999999998579 ) ) ;
#12180=EDGE_CURVE ( 'NONE', #1999, #13850, #8940, .T. ) ;
#12182=CARTESIAN_POINT ( 'NONE',  ( -30.00000000000000000, -42.57363661491096707, -121.3828884801879155 ) ) ;
#12184=DIRECTION ( 'NONE',  ( -1.000000000000000000, 0.000000000000000000, 0.000000000000000000 ) ) ;
#12193=DIRECTION ( 'NONE',  ( -0.000000000000000000, -1.000000000000000000, -0.000000000000000000 ) ) ;
#12198=DIRECTION ( 'NONE',  ( -1.000000000000000000, 0.000000000000000000, 0.000000000000000000 ) ) ;
#12201=DIRECTION ( 'NONE',  ( 0.000000000000000000, 0.000000000000000000, -1.000000000000000000 ) ) ;
#12204=ORIENTED_EDGE ( 'NONE', *, *, #672, .T. ) ;
#12206=EDGE_CURVE ( 'NONE', #10337, #7685, #4809, .T. ) ;
#12207=ORIENTED_EDGE ( 'NONE', *, *, #12871, .F. ) ;
#12209=CARTESIAN_POINT ( 'NONE',  ( -14.94551481348182165, -15.47228562136404584, 73.52041642655926523 ) ) ;
#12231=CARTESIAN_POINT ( 'NONE',  ( 9.482998254698379981, -19.29932845388887230, -71.54974094241291027 ) ) ;
#12234=CARTESIAN_POINT ( 'NONE',  ( -24.99999999999999289, -42.57363661491096707, -121.3828884801879155 ) ) ;
#12239=FACE_OUTER_BOUND ( 'NONE', #12985, .T. ) ;
#12247=DIRECTION ( 'NONE',  ( -1.000000000000000000, -0.000000000000000000, -0.000000000000000000 ) ) ;
#12253=AXIS2_PLACEMENT_3D ( 'NONE', #8054, #14422, #11226 ) ;
#12254=ORIENTED_EDGE ( 'NONE', *, *, #17922, .T. ) ;
#12255=CARTESIAN_POINT ( 'NONE',  ( -19.10408208028293586, -9.878941057108505674, 83.54765472770249346 ) ) ;
#12263=VECTOR ( 'NONE', #14198, 1000.000000000000000 ) ;
#12271=ORIENTED_EDGE ( 'NONE', *, *, #3009, .T. ) ;
#12273=ORIENTED_EDGE ( 'NONE', *, *, #13538, .F. ) ;
#12282=EDGE_LOOP ( 'NONE', ( #12624, #1543 ) ) ;
#12284=DIRECTION ( 'NONE',  ( 0.000000000000000000, 0.000000000000000000, -1.000000000000000000 ) ) ;
#12285=VECTOR ( 'NONE', #5159, 1000.000000000000000 ) ;
#12289=CARTESIAN_POINT ( 'NONE',  ( -27.96694501150314593, -24.74873734152930993, -120.0000000000000142 ) ) ;
#12293=DIRECTION ( 'NONE',  ( 1.000000000000000000, 0.000000000000000000, 0.000000000000000000 ) ) ;
#12296=AXIS2_PLACEMENT_3D ( 'NONE', #8791, #11875, #8699 ) ;
#12298=EDGE_LOOP ( 'NONE', ( #2463, #18389, #20453, #1995 ) ) ;
#12304=CIRCLE ( 'NONE', #7201, 35.00000000000000000 ) ;
#12306=DIRECTION ( 'NONE',  ( 0.000000000000000000, -0.000000000000000000, 1.000000000000000000 ) ) ;
#12313=CARTESIAN_POINT ( 'NONE',  ( 50.00000000000000000, -42.57363661491096707, -71.38288848018790134 ) ) ;
#12317=EDGE_CURVE ( 'NONE', #5157, #3526, #13692, .T. ) ;
#12318=AXIS2_PLACEMENT_3D ( 'NONE', #6779, #20127, #3911 ) ;
#12321=DIRECTION ( 'NONE',  ( 0.000000000000000000, 0.000000000000000000, -1.000000000000000000 ) ) ;
#12325=ORIENTED_EDGE ( 'NONE', *, *, #4138, .T. ) ;
#12328=CARTESIAN_POINT ( 'NONE',  ( 45.02826274242529081, -126.4302678889703202, 84.01931467314857116 ) ) ;
#12332=ORIENTED_EDGE ( 'NONE', *, *, #12480, .T. ) ;
#12333=LINE ( 'NONE', #18799, #2571 ) ;
#12335=CARTESIAN_POINT ( 'NONE',  ( 47.57345354676048998, -5.300163754693023144, 88.03325769612197860 ) ) ;
#12337=CARTESIAN_POINT ( 'NONE',  ( 49.19234958605026264, -1.326995226329893862, 84.99999999999998579 ) ) ;
#12357=AXIS2_PLACEMENT_3D ( 'NONE', #20675, #2678, #17204 ) ;
#12358=CARTESIAN_POINT ( 'NONE',  ( 24.99999999999999645, -110.0000000000000142, -45.00000000000000711 ) ) ;
#12359=B_SPLINE_CURVE_WITH_KNOTS ( 'NONE', 3,
 ( #15684, #13890, #11020, #11128, #17497, #9530, #1186, #6041, #18977, #12514, #20335, #7629, #10915, #14109, #20563, #4447, #17390, #3178, #15999, #19488, #16210, #1794 ),
 .UNSPECIFIED., .F., .F.,
 ( 4, 2, 2, 2, 2, 2, 2, 2, 2, 2, 4 ),
 ( 0.007433635558789152172, 0.01246066521146292627, 0.01497418003779982937, 0.01748769486413673246, 0.02754175416948434832, 0.03005526899582125142, 0.03256878382215815798, 0.03759581347483195030, 0.04262284312750573567, 0.04513635795384261795, 0.04764987278017949329 ),
 .UNSPECIFIED. ) ;
#12360=EDGE_CURVE ( 'NONE', #3206, #17908, #8662, .T. ) ;
#12361=ORIENTED_EDGE ( 'NONE', *, *, #15051, .F. ) ;
#12363=CARTESIAN_POINT ( 'NONE',  ( 30.25309211476868398, -108.6363473640507920, 73.18580831706346146 ) ) ;
#12364=ADVANCED_FACE ( 'NONE', ( #10741 ), #4469, .T. ) ;
#12368=ORIENTED_EDGE ( 'NONE', *, *, #17213, .T. ) ;
#12371=CARTESIAN_POINT ( 'NONE',  ( -18.83539447212728390, -10.38388837219175542, 83.11735093927855189 ) ) ;
#12374=DIRECTION ( 'NONE',  ( 0.000000000000000000, 0.000000000000000000, 1.000000000000000000 ) ) ;
#12378=ORIENTED_EDGE ( 'NONE', *, *, #18666, .T. ) ;
#12381=DIRECTION ( 'NONE',  ( 1.000000000000000000, 0.000000000000000000, 0.000000000000000000 ) ) ;
#12385=CARTESIAN_POINT ( 'NONE',  ( 10.00000000000000178, -164.9999999999999716, 70.00000000000000000 ) ) ;
#12390=UNCERTAINTY_MEASURE_WITH_UNIT (LENGTH_MEASURE( 1.000000000000000082E-05 ), #1927, 'distance_accuracy_value', 'NONE');
#12391=VECTOR ( 'NONE', #2725, 1000.000000000000114 ) ;
#12407=DIRECTION ( 'NONE',  ( 1.000000000000000000, 0.000000000000000000, 0.000000000000000000 ) ) ;
#12417=PLANE ( 'NONE',  #13940 ) ;
#12420=EDGE_CURVE ( 'NONE', #18257, #15415, #10666, .T. ) ;
#12422=DIRECTION ( 'NONE',  ( -0.000000000000000000, -0.000000000000000000, 1.000000000000000000 ) ) ;
#12423=FACE_BOUND ( 'NONE', #2786, .T. ) ;
#12432=EDGE_CURVE ( 'NONE', #5100, #12774, #6920, .T. ) ;
#12434=VERTEX_POINT ( 'NONE', #7650 ) ;
#12447=ORIENTED_EDGE ( 'NONE', *, *, #1219, .T. ) ;
#12457=CARTESIAN_POINT ( 'NONE',  ( 30.00000000000000000, -39.99999999999999289, 49.90000000000000568 ) ) ;
#12458=DIRECTION ( 'NONE',  ( 0.000000000000000000, 0.000000000000000000, -1.000000000000000000 ) ) ;
#12461=AXIS2_PLACEMENT_3D ( 'NONE', #19474, #3361, #185 ) ;
#12463=VERTEX_POINT ( 'NONE', #12756 ) ;
#12464=CARTESIAN_POINT ( 'NONE',  ( 29.99999999999965183, -164.9999999999999716, -50.00000000000002842 ) ) ;
#12466=ORIENTED_EDGE ( 'NONE', *, *, #668, .F. ) ;
#12468=EDGE_CURVE ( 'NONE', #18656, #4973, #16073, .T. ) ;
#12469=CARTESIAN_POINT ( 'NONE',  ( 31.27523735953079864, -112.0413217638139827, 74.38135980682834258 ) ) ;
#12475=CARTESIAN_POINT ( 'NONE',  ( 18.21773432164967232, -11.43289491867056817, 82.25893718214402384 ) ) ;
#12480=EDGE_CURVE ( 'NONE', #9722, #8274, #14027, .T. ) ;
#12484=CARTESIAN_POINT ( 'NONE',  ( 30.00000000000000355, -139.6410161513775563, 90.00000000000001421 ) ) ;
#12487=CARTESIAN_POINT ( 'NONE',  ( 19.58689223458519990, -12.07292356518670395, -81.75718538670371061 ) ) ;
#12492=ORIENTED_EDGE ( 'NONE', *, *, #7392, .F. ) ;
#12500=VERTEX_POINT ( 'NONE', #6466 ) ;
#12503=EDGE_CURVE ( 'NONE', #15865, #11773, #6777, .T. ) ;
#12513=ORIENTED_EDGE ( 'NONE', *, *, #3660, .F. ) ;
#12514=CARTESIAN_POINT ( 'NONE',  ( 36.05404575234035747, -22.88198422515676356, -75.41713818884518616 ) ) ;
#12518=CARTESIAN_POINT ( 'NONE',  ( 30.00000000000000000, -105.0000000000000000, -72.35596062816881613 ) ) ;
#12519=ADVANCED_FACE ( 'NONE', ( #16427 ), #9668, .T. ) ;
#12523=DIRECTION ( 'NONE',  ( 1.000000000000000000, 0.000000000000000000, 0.000000000000000000 ) ) ;
#12529=DIRECTION ( 'NONE',  ( 0.000000000000000000, 0.000000000000000000, -1.000000000000000000 ) ) ;
#12533=ORIENTED_EDGE ( 'NONE', *, *, #18675, .T. ) ;
#12539=CIRCLE ( 'NONE', #17289, 8.500000000000000000 ) ;
#12542=EDGE_CURVE ( 'NONE', #5755, #12500, #5191, .T. ) ;
#12548=ORIENTED_EDGE ( 'NONE', *, *, #6048, .T. ) ;
#12553=LINE ( 'NONE', #19017, #4184 ) ;
#12559=VERTEX_POINT ( 'NONE', #14848 ) ;
#12560=CARTESIAN_POINT ( 'NONE',  ( 30.43430782549248903, -42.57363661491096707, -66.38288848018790134 ) ) ;
#12566=CARTESIAN_POINT ( 'NONE',  ( 30.00000000000000000, -106.8560220274159178, 72.71043371383413501 ) ) ;
#12570=EDGE_CURVE ( 'NONE', #14189, #17002, #19609, .T. ) ;
#12575=CARTESIAN_POINT ( 'NONE',  ( 20.81358546886585970, -5.482701416275067352, 87.82403804495045563 ) ) ;
#12582=ORIENTED_EDGE ( 'NONE', *, *, #3284, .T. ) ;
#12586=CARTESIAN_POINT ( 'NONE',  ( -15.15258959384416393, -17.31827655254226528, -78.22681860575444546 ) ) ;
#12587=CARTESIAN_POINT ( 'NONE',  ( 40.00000000000000711, -122.3205080756887781, -90.00000000000001421 ) ) ;
#12596=CARTESIAN_POINT ( 'NONE',  ( 0.000000000000000000, 0.000000000000000000, -130.0000000000000000 ) ) ;
#12600=EDGE_CURVE ( 'NONE', #14667, #18686, #14548, .T. ) ;
#12604=AXIS2_PLACEMENT_3D ( 'NONE', #2730, #10893, #17367 ) ;
#12607=EDGE_CURVE ( 'NONE', #13795, #8249, #17726, .T. ) ;
#12609=EDGE_CURVE ( 'NONE', #10422, #20655, #15382, .T. ) ;
#12611=VECTOR ( 'NONE', #16533, 1000.000000000000000 ) ;
#12613=CIRCLE ( 'NONE', #6171, 75.00000000000000000 ) ;
#12616=CARTESIAN_POINT ( 'NONE',  ( 30.43430782549247837, -42.57363661491096707, -71.38288848018790134 ) ) ;
#12618=ORIENTED_EDGE ( 'NONE', *, *, #14250, .T. ) ;
#12619=DIRECTION ( 'NONE',  ( -0.000000000000000000, -0.000000000000000000, 1.000000000000000000 ) ) ;
#12620=ORIENTED_EDGE ( 'NONE', *, *, #14658, .F. ) ;
#12621=ADVANCED_FACE ( 'NONE', ( #19405 ), #4893, .T. ) ;
#12624=ORIENTED_EDGE ( 'NONE', *, *, #6397, .F. ) ;
#12626=VERTEX_POINT ( 'NONE', #9766 ) ;
#12627=CARTESIAN_POINT ( 'NONE',  ( 31.94823399543905040, -113.6545208995224954, -75.04431888125806438 ) ) ;
#12648=VECTOR ( 'NONE', #7585, 1000.000000000000000 ) ;
#12663=DIRECTION ( 'NONE',  ( 0.000000000000000000, 0.000000000000000000, 1.000000000000000000 ) ) ;
#12668=DIRECTION ( 'NONE',  ( 0.000000000000000000, -8.673617379884036705E-17, 1.000000000000000000 ) ) ;
#12670=ADVANCED_FACE ( 'NONE', ( #16535 ), #8581, .F. ) ;
#12671=ORIENTED_EDGE ( 'NONE', *, *, #15716, .T. ) ;
#12675=DIRECTION ( 'NONE',  ( -1.000000000000000000, 0.000000000000000000, 0.000000000000000000 ) ) ;
#12682=ORIENTED_EDGE ( 'NONE', *, *, #3910, .F. ) ;
#12683=AXIS2_PLACEMENT_3D ( 'NONE', #12880, #14669, #19632 ) ;
#12691=CARTESIAN_POINT ( 'NONE',  ( -30.00000000000000000, -151.4095880458873467, -44.60680010464253087 ) ) ;
#12692=ORIENTED_EDGE ( 'NONE', *, *, #296, .F. ) ;
#12693=CARTESIAN_POINT ( 'NONE',  ( 2.822967073032372820, -21.36251226604836617, 76.10389727344437460 ) ) ;
#12697=DIRECTION ( 'NONE',  ( -0.000000000000000000, 0.7812527682501551052, 0.6242147964454779485 ) ) ;
#12699=DIRECTION ( 'NONE',  ( 0.000000000000000000, 0.000000000000000000, -1.000000000000000000 ) ) ;
#12703=EDGE_CURVE ( 'NONE', #12774, #17279, #11770, .T. ) ;
#12705=DIRECTION ( 'NONE',  ( 0.000000000000000000, 0.000000000000000000, -1.000000000000000000 ) ) ;
#12709=CIRCLE ( 'NONE', #1550, 205.0000000000000284 ) ;
#12712=ADVANCED_FACE ( 'NONE', ( #13368 ), #13676, .F. ) ;
#12723=ORIENTED_EDGE ( 'NONE', *, *, #16095, .T. ) ;
#12726=CARTESIAN_POINT ( 'NONE',  ( 30.02285928914783142, -48.02662919861900548, 66.64486488415462873 ) ) ;
#12731=DIRECTION ( 'NONE',  ( -0.000000000000000000, -0.000000000000000000, 1.000000000000000000 ) ) ;
#12734=VERTEX_POINT ( 'NONE', #15255 ) ;
#12739=ADVANCED_FACE ( 'NONE', ( #10078, #16948, #2123, #8896, #2019, #15056 ), #429, .T. ) ;
#12753=VECTOR ( 'NONE', #8592, 1000.000000000000000 ) ;
#12754=ORIENTED_EDGE ( 'NONE', *, *, #9539, .F. ) ;
#12756=CARTESIAN_POINT ( 'NONE',  ( 30.00000000000000000, -30.00000000000000711, 44.99999999999998579 ) ) ;
#12757=EDGE_LOOP ( 'NONE', ( #10837, #5663 ) ) ;
#12758=CARTESIAN_POINT ( 'NONE',  ( -22.70866746290765903, -3.649167310370807105, -90.00000000000000000 ) ) ;
#12763=DIRECTION ( 'NONE',  ( 0.000000000000000000, -0.000000000000000000, 1.000000000000000000 ) ) ;
#12766=ORIENTED_EDGE ( 'NONE', *, *, #12609, .F. ) ;
#12774=VERTEX_POINT ( 'NONE', #7831 ) ;
#12778=ORIENTED_EDGE ( 'NONE', *, *, #554, .T. ) ;
#12782=VERTEX_POINT ( 'NONE', #10909 ) ;
#12784=CARTESIAN_POINT ( 'NONE',  ( 21.50000000000000000, 2.632990618166809235E-15, -68.00000000000000000 ) ) ;
#12786=AXIS2_PLACEMENT_3D ( 'NONE', #2549, #14105, #20558 ) ;
#12787=ORIENTED_EDGE ( 'NONE', *, *, #8367, .F. ) ;
#12788=CARTESIAN_POINT ( 'NONE',  ( -30.00000000000000000, 36.35083268962915781, -50.00000000000000000 ) ) ;
#12789=EDGE_LOOP ( 'NONE', ( #823, #6157 ) ) ;
#12792=ORIENTED_EDGE ( 'NONE', *, *, #6389, .F. ) ;
#12802=CARTESIAN_POINT ( 'NONE',  ( 30.00000000000000000, -110.0000000000000000, -45.00000000000000711 ) ) ;
#12812=ORIENTED_EDGE ( 'NONE', *, *, #12360, .F. ) ;
#12813=CARTESIAN_POINT ( 'NONE',  ( -18.07215471859532485, -14.28798666575421628, -80.13107141598003125 ) ) ;
#12817=CARTESIAN_POINT ( 'NONE',  ( 43.62500077266424370, -124.9999999999999858, -90.00000000000001421 ) ) ;
#12823=DIRECTION ( 'NONE',  ( -1.000000000000000000, -0.000000000000000000, -0.000000000000000000 ) ) ;
#12825=EDGE_CURVE ( 'NONE', #18745, #19852, #13116, .T. ) ;
#12827=CARTESIAN_POINT ( 'NONE',  ( 42.61160110135222823, -124.0569253416645523, -88.80170281571382418 ) ) ;
#12831=CARTESIAN_POINT ( 'NONE',  ( 36.91783118030027566, -21.11288316874070858, 70.73473707049505776 ) ) ;
#12841=CARTESIAN_POINT ( 'NONE',  ( 0.000000000000000000, 0.000000000000000000, -90.00000000000000000 ) ) ;
#12849=DIRECTION ( 'NONE',  ( 0.000000000000000000, 0.000000000000000000, -1.000000000000000000 ) ) ;
#12855=EDGE_CURVE ( 'NONE', #2608, #20537, #7619, .T. ) ;
#12860=CARTESIAN_POINT ( 'NONE',  ( 31.48871417509230142, -36.16658848463109166, 71.75696761739389729 ) ) ;
#12865=ADVANCED_FACE ( 'NONE', ( #9323 ), #6134, .F. ) ;
#12866=FACE_BOUND ( 'NONE', #5908, .T. ) ;
#12871=EDGE_CURVE ( 'NONE', #3436, #1656, #17861, .T. ) ;
#12876=ADVANCED_FACE ( 'NONE', ( #10603 ), #13995, .F. ) ;
#12879=DIRECTION ( 'NONE',  ( -1.000000000000000000, 0.000000000000000000, 0.000000000000000000 ) ) ;
#12880=CARTESIAN_POINT ( 'NONE',  ( 0.000000000000000000, 0.000000000000000000, -81.99999999999998579 ) ) ;
#12883=ORIENTED_EDGE ( 'NONE', *, *, #12420, .T. ) ;
#12890=VECTOR ( 'NONE', #8105, 1000.000000000000000 ) ;
#12892=ORIENTED_EDGE ( 'NONE', *, *, #16469, .F. ) ;
#12895=CARTESIAN_POINT ( 'NONE',  ( 50.00000000000000000, -124.9999999999999858, -90.00000000000001421 ) ) ;
#12898=CARTESIAN_POINT ( 'NONE',  ( 10.00000000000000178, -160.0000000000000000, -70.00000000000000000 ) ) ;
#12901=VERTEX_POINT ( 'NONE', #18875 ) ;
#12906=VERTEX_POINT ( 'NONE', #19274 ) ;
#12910=DIRECTION ( 'NONE',  ( 0.000000000000000000, -0.000000000000000000, -1.000000000000000000 ) ) ;
#12914=ORIENTED_EDGE ( 'NONE', *, *, #6737, .F. ) ;
#12919=FACE_OUTER_BOUND ( 'NONE', #3086, .T. ) ;
#12932=LINE ( 'NONE', #9748, #4462 ) ;
#12946=AXIS2_PLACEMENT_3D ( 'NONE', #15162, #16638, #14954 ) ;
#12953=DIRECTION ( 'NONE',  ( 0.000000000000000000, 0.000000000000000000, -1.000000000000000000 ) ) ;
#12961=LINE ( 'NONE', #3502, #13071 ) ;
#12967=LINE ( 'NONE', #6694, #20767 ) ;
#12969=EDGE_LOOP ( 'NONE', ( #3782, #13078, #8390, #3091 ) ) ;
#12979=DIRECTION ( 'NONE',  ( -1.000000000000000000, 0.000000000000000000, 0.000000000000000000 ) ) ;
#12980=ORIENTED_EDGE ( 'NONE', *, *, #7907, .T. ) ;
#12982=VERTEX_POINT ( 'NONE', #6242 ) ;
#12985=EDGE_LOOP ( 'NONE', ( #18903, #15612, #2357, #11690, #15108, #17950, #20122, #11841, #16639, #10281, #12466, #11725, #18232, #15497 ) ) ;
#12986=ADVANCED_FACE ( 'NONE', ( #6655 ), #9525, .T. ) ;
#12990=EDGE_CURVE ( 'NONE', #7867, #13475, #3275, .T. ) ;
#13003=EDGE_CURVE ( 'NONE', #9313, #8953, #11416, .T. ) ;
#13007=ORIENTED_EDGE ( 'NONE', *, *, #2852, .T. ) ;
#13021=VECTOR ( 'NONE', #11661, 1000.000000000000000 ) ;
#13025=ORIENTED_EDGE ( 'NONE', *, *, #1359, .T. ) ;
#13026=VERTEX_POINT ( 'NONE', #3772 ) ;
#13034=CYLINDRICAL_SURFACE ( 'NONE', #6481, 80.00000000000000000 ) ;
#13036=ORIENTED_EDGE ( 'NONE', *, *, #7007, .T. ) ;
#13042=CARTESIAN_POINT ( 'NONE',  ( -24.99999999999999289, 31.35083268962915426, 84.99999999999998579 ) ) ;
#13048=CARTESIAN_POINT ( 'NONE',  ( 50.00000000000000000, -105.0000000000000284, -77.45966692414833688 ) ) ;
#13057=DIRECTION ( 'NONE',  ( 0.000000000000000000, 0.000000000000000000, -1.000000000000000000 ) ) ;
#13059=AXIS2_PLACEMENT_3D ( 'NONE', #6732, #14596, #13114 ) ;
#13063=VECTOR ( 'NONE', #20469, 1000.000000000000000 ) ;
#13065=SURFACE_STYLE_FILL_AREA ( #9974 ) ;
#13071=VECTOR ( 'NONE', #1827, 1000.000000000000000 ) ;
#13074=CYLINDRICAL_SURFACE ( 'NONE', #8573, 2.099999999999997868 ) ;
#13076=AXIS2_PLACEMENT_3D ( 'NONE', #15520, #906, #13837 ) ;
#13078=ORIENTED_EDGE ( 'NONE', *, *, #16005, .T. ) ;
#13082=DIRECTION ( 'NONE',  ( -0.000000000000000000, -1.000000000000000000, -0.000000000000000000 ) ) ;
#13096=CARTESIAN_POINT ( 'NONE',  ( 24.99999999999999645, -122.0000000000000000, -6.368163355566234804E-15 ) ) ;
#13100=FACE_OUTER_BOUND ( 'NONE', #2590, .T. ) ;
#13101=EDGE_CURVE ( 'NONE', #20455, #7012, #16957, .T. ) ;
#13114=DIRECTION ( 'NONE',  ( 0.000000000000000000, 0.000000000000000000, -1.000000000000000000 ) ) ;
#13116=CIRCLE ( 'NONE', #16498, 50.00000000000001421 ) ;
#13119=AXIS2_PLACEMENT_3D ( 'NONE', #20926, #4819, #3027 ) ;
#13123=EDGE_CURVE ( 'NONE', #1189, #10440, #3676, .T. ) ;
#13137=CIRCLE ( 'NONE', #4674, 2.099999999999997868 ) ;
#13138=CARTESIAN_POINT ( 'NONE',  ( 30.00000000000000000, -85.00000000000000000, -1.040949779275250179E-14 ) ) ;
#13139=CARTESIAN_POINT ( 'NONE',  ( 34.94904587705838850, -25.30803235969634457, 69.13077653488730334 ) ) ;
#13140=VERTEX_POINT ( 'NONE', #2523 ) ;
#13143=FACE_BOUND ( 'NONE', #1719, .T. ) ;
#13144=DIRECTION ( 'NONE',  ( 1.000000000000000000, 0.000000000000000000, 0.000000000000000000 ) ) ;
#13149=DIRECTION ( 'NONE',  ( 1.000000000000000000, 0.000000000000000000, 0.000000000000000000 ) ) ;
#13155=CYLINDRICAL_SURFACE ( 'NONE', #14433, 2.099999999999997868 ) ;
#13160=VERTEX_POINT ( 'NONE', #7381 ) ;
#13169=CARTESIAN_POINT ( 'NONE',  ( 30.00000000000000000, -99.99999999999998579, 52.00000000000000000 ) ) ;
#13175=CARTESIAN_POINT ( 'NONE',  ( 30.00000000000000000, -105.0000000000000000, -77.45966692414833688 ) ) ;
#13176=SURFACE_STYLE_USAGE ( .BOTH. , #13583 ) ;
#13177=CARTESIAN_POINT ( 'NONE',  ( -44.00000000000000000, -85.00000000000000000, 14.49999999999998579 ) ) ;
#13179=VECTOR ( 'NONE', #1619, 1000.000000000000000 ) ;
#13181=CARTESIAN_POINT ( 'NONE',  ( -24.99999999999999289, -85.00000000000000000, -1.040949779275250179E-14 ) ) ;
#13184=CARTESIAN_POINT ( 'NONE',  ( -44.00000000000000000, -85.00000000000000000, -1.040949779275250179E-14 ) ) ;
#13185=ORIENTED_EDGE ( 'NONE', *, *, #19984, .F. ) ;
#13186=FACE_OUTER_BOUND ( 'NONE', #20257, .T. ) ;
#13187=VERTEX_POINT ( 'NONE', #20206 ) ;
#13190=ADVANCED_FACE ( 'NONE', ( #8980 ), #4417, .F. ) ;
#13193=CARTESIAN_POINT ( 'NONE',  ( -24.99999999999999289, -85.00000000000000000, -1.040949779275250179E-14 ) ) ;
#13199=CARTESIAN_POINT ( 'NONE',  ( 0.000000000000000000, 0.000000000000000000, -90.00000000000000000 ) ) ;
#13206=EDGE_LOOP ( 'NONE', ( #17943, #3397, #7579, #7879 ) ) ;
#13213=DIRECTION ( 'NONE',  ( 0.000000000000000000, 0.000000000000000000, -1.000000000000000000 ) ) ;
#13225=EDGE_LOOP ( 'NONE', ( #8378, #8720 ) ) ;
#13226=VECTOR ( 'NONE', #6163, 1000.000000000000000 ) ;
#13234=DIRECTION ( 'NONE',  ( 0.000000000000000000, 0.000000000000000000, -1.000000000000000000 ) ) ;
#13235=DIRECTION ( 'NONE',  ( 0.000000000000000000, 0.000000000000000000, -1.000000000000000000 ) ) ;
#13238=CARTESIAN_POINT ( 'NONE',  ( -24.99999999999999289, 31.35083268962915426, 50.63110039191614220 ) ) ;
#13240=EDGE_CURVE ( 'NONE', #11744, #11554, #6343, .T. ) ;
#13253=EDGE_CURVE ( 'NONE', #20655, #10422, #8046, .T. ) ;
#13254=EDGE_LOOP ( 'NONE', ( #17092, #13944, #7942, #7416 ) ) ;
#13260=ORIENTED_EDGE ( 'NONE', *, *, #6737, .T. ) ;
#13262=DIRECTION ( 'NONE',  ( 1.000000000000000000, -0.000000000000000000, -0.000000000000000000 ) ) ;
#13263=VERTEX_POINT ( 'NONE', #20630 ) ;
#13271=VECTOR ( 'NONE', #11084, 1000.000000000000000 ) ;
#13274=AXIS2_PLACEMENT_3D ( 'NONE', #15682, #6136, #12184 ) ;
#13279=DIRECTION ( 'NONE',  ( 0.000000000000000000, 0.000000000000000000, -1.000000000000000000 ) ) ;
#13280=VERTEX_POINT ( 'NONE', #17674 ) ;
#13285=VECTOR ( 'NONE', #20317, 1000.000000000000000 ) ;
#13289=ORIENTED_EDGE ( 'NONE', *, *, #20113, .F. ) ;
#13292=AXIS2_PLACEMENT_3D ( 'NONE', #9507, #7920, #376 ) ;
#13294=CIRCLE ( 'NONE', #7531, 5.000000000000004441 ) ;
#13301=ORIENTED_EDGE ( 'NONE', *, *, #2945, .F. ) ;
#13302=DIRECTION ( 'NONE',  ( 0.000000000000000000, 0.000000000000000000, 1.000000000000000000 ) ) ;
#13304=EDGE_CURVE ( 'NONE', #3394, #10440, #1466, .T. ) ;
#13306=AXIS2_PLACEMENT_3D ( 'NONE', #12033, #15213, #20077 ) ;
#13311=CARTESIAN_POINT ( 'NONE',  ( -30.00000000000000000, -164.9999999999999716, 90.00000000000001421 ) ) ;
#13313=AXIS2_PLACEMENT_3D ( 'NONE', #11639, #8146, #16111 ) ;
#13314=AXIS2_PLACEMENT_3D ( 'NONE', #9537, #17400, #4568 ) ;
#13320=AXIS2_PLACEMENT_3D ( 'NONE', #14773, #18059, #8198 ) ;
#13331=AXIS2_PLACEMENT_3D ( 'NONE', #19620, #16341, #336 ) ;
#13336=ADVANCED_FACE ( 'NONE', ( #10107, #11589 ), #9615, .F. ) ;
#13338=EDGE_LOOP ( 'NONE', ( #19004, #20710, #2278, #3760, #12812, #5063 ) ) ;
#13340=CARTESIAN_POINT ( 'NONE',  ( 45.76122707727121508, -127.3290820621008947, -85.00000000000000000 ) ) ;
#13345=ORIENTED_EDGE ( 'NONE', *, *, #1087, .T. ) ;
#13348=ORIENTED_EDGE ( 'NONE', *, *, #3009, .F. ) ;
#13356=DIRECTION ( 'NONE',  ( 0.000000000000000000, 0.000000000000000000, 1.000000000000000000 ) ) ;
#13365=CARTESIAN_POINT ( 'NONE',  ( 24.99999999999999645, -99.99999999999998579, -54.09999999999999432 ) ) ;
#13368=FACE_OUTER_BOUND ( 'NONE', #1712, .T. ) ;
#13370=CYLINDRICAL_SURFACE ( 'NONE', #807, 2.099999999999997868 ) ;
#13375=ORIENTED_EDGE ( 'NONE', *, *, #296, .T. ) ;
#13376=EDGE_CURVE ( 'NONE', #17173, #5499, #8500, .T. ) ;
#13381=CARTESIAN_POINT ( 'NONE',  ( -26.35784117651625280, 26.35784117651607872, -120.0000000000000142 ) ) ;
#13387=CARTESIAN_POINT ( 'NONE',  ( 39.25023869350728489, -121.8876331835572415, -86.53734499821167958 ) ) ;
#13390=LINE ( 'NONE', #13808, #6451 ) ;
#13397=CARTESIAN_POINT ( 'NONE',  ( -21.25952603694473808, -3.390848217253790597, 82.75718265314236533 ) ) ;
#13398=ORIENTED_EDGE ( 'NONE', *, *, #166, .T. ) ;
#13417=CARTESIAN_POINT ( 'NONE',  ( -21.39626923676110337, -2.341574137301850822, -83.84978971573227113 ) ) ;
#13424=ORIENTED_EDGE ( 'NONE', *, *, #9374, .T. ) ;
#13425=CYLINDRICAL_SURFACE ( 'NONE', #446, 21.50000000000000000 ) ;
#13433=LINE ( 'NONE', #16699, #2799 ) ;
#13439=ORIENTED_EDGE ( 'NONE', *, *, #3243, .T. ) ;
#13442=COLOUR_RGB ( '', 0.66274510, 0.83137255, 0.94901961) ;
#13443=DIRECTION ( 'NONE',  ( 0.000000000000000000, 0.000000000000000000, -1.000000000000000000 ) ) ;
#13447=AXIS2_PLACEMENT_3D ( 'NONE', #1289, #18768, #4236 ) ;
#13456=FACE_OUTER_BOUND ( 'NONE', #9084, .T. ) ;
#13459=DIRECTION ( 'NONE',  ( 0.000000000000000000, 0.000000000000000000, 1.000000000000000000 ) ) ;
#13474=DIRECTION ( 'NONE',  ( 1.000000000000000000, 0.000000000000000000, -0.000000000000000000 ) ) ;
#13475=VERTEX_POINT ( 'NONE', #996 ) ;
#13476=CARTESIAN_POINT ( 'NONE',  ( 50.00000000000000000, -164.9999999999999716, -90.00000000000001421 ) ) ;
#13480=ORIENTED_EDGE ( 'NONE', *, *, #4017, .F. ) ;
#13481=ORIENTED_EDGE ( 'NONE', *, *, #803, .T. ) ;
#13482=LINE ( 'NONE', #20246, #3583 ) ;
#13483=CARTESIAN_POINT ( 'NONE',  ( 48.35276434571220250, -3.649167310370807105, -90.00000000000000000 ) ) ;
#13484=EDGE_CURVE ( 'NONE', #18682, #2149, #5855, .T. ) ;
#13490=DIRECTION ( 'NONE',  ( -1.000000000000000000, 0.000000000000000000, 0.000000000000000000 ) ) ;
#13493=ORIENTED_EDGE ( 'NONE', *, *, #6048, .F. ) ;
#13494=LINE ( 'NONE', #19936, #2097 ) ;
#13497=CARTESIAN_POINT ( 'NONE',  ( -3.872723063507635732, -21.16211945945223505, 70.72147569179593063 ) ) ;
#13503=ORIENTED_EDGE ( 'NONE', *, *, #1348, .F. ) ;
#13513=ORIENTED_EDGE ( 'NONE', *, *, #14886, .F. ) ;
#13514=CARTESIAN_POINT ( 'NONE',  ( 50.00000000000000000, -42.57363661491096707, -121.3828884801879155 ) ) ;
#13516=CARTESIAN_POINT ( 'NONE',  ( -9.249412617561571182, -19.41235462500714348, -71.49717528132289601 ) ) ;
#13519=DIRECTION ( 'NONE',  ( 1.000000000000000000, 0.000000000000000000, 0.000000000000000000 ) ) ;
#13520=DIRECTION ( 'NONE',  ( 0.000000000000000000, 0.000000000000000000, 1.000000000000000000 ) ) ;
#13524=ORIENTED_EDGE ( 'NONE', *, *, #6652, .F. ) ;
#13528=DIRECTION ( 'NONE',  ( -0.000000000000000000, -0.000000000000000000, 1.000000000000000000 ) ) ;
#13529=ADVANCED_FACE ( 'NONE', ( #4046 ), #11894, .T. ) ;
#13538=EDGE_CURVE ( 'NONE', #15733, #18615, #3833, .T. ) ;
#13541=CARTESIAN_POINT ( 'NONE',  ( 33.05360093408142319, -115.6303066365226471, 81.70693292403575470 ) ) ;
#13542=CARTESIAN_POINT ( 'NONE',  ( 45.06005321672401465, -126.4314683844613683, -83.99502465749384328 ) ) ;
#13548=ORIENTED_EDGE ( 'NONE', *, *, #18009, .F. ) ;
#13553=CARTESIAN_POINT ( 'NONE',  ( -30.00000000000000000, -40.00000000000000000, -120.0000000000000142 ) ) ;
#13572=CARTESIAN_POINT ( 'NONE',  ( 41.63608460325703220, -13.17366712949431218, -74.81088764122226564 ) ) ;
#13576=CYLINDRICAL_SURFACE ( 'NONE', #8324, 39.99999999999999289 ) ;
#13581=DIRECTION ( 'NONE',  ( 1.000000000000000000, -0.000000000000000000, -0.000000000000000000 ) ) ;
#13583=SURFACE_SIDE_STYLE ('',( #10304 ) ) ;
#13590=CARTESIAN_POINT ( 'NONE',  ( 11.44271251907791154, -18.21718295280816236, 72.06823551977507236 ) ) ;
#13595=ORIENTED_EDGE ( 'NONE', *, *, #9254, .T. ) ;
#13600=CIRCLE ( 'NONE', #15976, 75.00000000000001421 ) ;
#13602=CARTESIAN_POINT ( 'NONE',  ( -24.99999999999999289, -160.0000000000000000, 0.000000000000000000 ) ) ;
#13613=CIRCLE ( 'NONE', #16999, 5.000000000000000888 ) ;
#13614=CARTESIAN_POINT ( 'NONE',  ( -19.43057967899846616, -9.208910241125160212, -77.65734690581830080 ) ) ;
#13619=CARTESIAN_POINT ( 'NONE',  ( 50.00000000000000000, -139.6410161513775563, 90.00000000000001421 ) ) ;
#13622=LINE ( 'NONE', #13840, #11272 ) ;
#13624=DIRECTION ( 'NONE',  ( 0.000000000000000000, 0.000000000000000000, -1.000000000000000000 ) ) ;
#13627=CARTESIAN_POINT ( 'NONE',  ( 30.00000000000000000, -85.00000000000000000, -1.040949779275250179E-14 ) ) ;
#13633=CARTESIAN_POINT ( 'NONE',  ( 30.00000000000001066, 39.99999999999998579, -130.0000000000000000 ) ) ;
#13636=EDGE_LOOP ( 'NONE', ( #11362, #6321, #6817, #19466 ) ) ;
#13640=CARTESIAN_POINT ( 'NONE',  ( -17.73632026622077618, -12.15589442372808548, 81.69840364569164137 ) ) ;
#13643=DIRECTION ( 'NONE',  ( 1.000000000000000000, -0.000000000000000000, -0.000000000000000000 ) ) ;
#13649=CARTESIAN_POINT ( 'NONE',  ( 41.19307857824662733, -123.0525692265442785, -80.87006134762231113 ) ) ;
#13651=CARTESIAN_POINT ( 'NONE',  ( 6.134128071782536828, -22.22025288403098386, -75.71173876110991330 ) ) ;
#13657=ORIENTED_EDGE ( 'NONE', *, *, #12871, .T. ) ;
#13666=DIRECTION ( 'NONE',  ( 0.000000000000000000, 1.040834085586084454E-15, -1.000000000000000000 ) ) ;
#13676=CYLINDRICAL_SURFACE ( 'NONE', #14478, 18.00000000000000000 ) ;
#13679=FACE_OUTER_BOUND ( 'NONE', #7598, .T. ) ;
#13682=FACE_OUTER_BOUND ( 'NONE', #20660, .T. ) ;
#13690=DIRECTION ( 'NONE',  ( 1.000000000000000000, 0.000000000000000000, -0.000000000000000000 ) ) ;
#13692=CIRCLE ( 'NONE', #19781, 200.0000000000000000 ) ;
#13697=ORIENTED_EDGE ( 'NONE', *, *, #13123, .F. ) ;
#13702=VERTEX_POINT ( 'NONE', #17210 ) ;
#13711=EDGE_CURVE ( 'NONE', #8274, #7282, #15603, .T. ) ;
#13712=DIRECTION ( 'NONE',  ( -0.000000000000000000, -0.000000000000000000, 1.000000000000000000 ) ) ;
#13718=EDGE_CURVE ( 'NONE', #5869, #20752, #18164, .T. ) ;
#13723=CARTESIAN_POINT ( 'NONE',  ( 14.60954982181485740, -15.77788197283119409, -73.35099031848521633 ) ) ;
#13725=ORIENTED_EDGE ( 'NONE', *, *, #10184, .T. ) ;
#13727=DIRECTION ( 'NONE',  ( -1.000000000000000000, 0.000000000000000000, 0.000000000000000000 ) ) ;
#13729=ORIENTED_EDGE ( 'NONE', *, *, #10184, .F. ) ;
#13730=FACE_BOUND ( 'NONE', #18605, .T. ) ;
#13734=DIRECTION ( 'NONE',  ( 0.000000000000000000, 0.000000000000000000, 1.000000000000000000 ) ) ;
#13736=DIRECTION ( 'NONE',  ( 0.000000000000000000, 0.000000000000000000, -1.000000000000000000 ) ) ;
#13741=EDGE_CURVE ( 'NONE', #5402, #4186, #3592, .T. ) ;
#13750=ADVANCED_FACE ( 'NONE', ( #15920 ), #2785, .T. ) ;
#13755=DIRECTION ( 'NONE',  ( 0.000000000000000000, -0.000000000000000000, 1.000000000000000000 ) ) ;
#13756=ORIENTED_EDGE ( 'NONE', *, *, #13864, .T. ) ;
#13764=DIRECTION ( 'NONE',  ( 0.000000000000000000, 0.000000000000000000, -1.000000000000000000 ) ) ;
#13770=DIRECTION ( 'NONE',  ( 0.000000000000000000, 0.000000000000000000, 1.000000000000000000 ) ) ;
#13790=CIRCLE ( 'NONE', #20201, 23.00000000000000000 ) ;
#13795=VERTEX_POINT ( 'NONE', #14643 ) ;
#13808=CARTESIAN_POINT ( 'NONE',  ( 30.00000000000001066, 39.99999999999998579, -120.0000000000000142 ) ) ;
#13812=DIRECTION ( 'NONE',  ( -1.000000000000000000, 0.000000000000000000, 0.000000000000000000 ) ) ;
#13815=CARTESIAN_POINT ( 'NONE',  ( 13.23800900960919158, -16.95692081615699820, 72.71034110640577808 ) ) ;
#13819=DIRECTION ( 'NONE',  ( 1.000000000000000000, 0.000000000000000000, 0.000000000000000000 ) ) ;
#13832=ORIENTED_EDGE ( 'NONE', *, *, #4791, .T. ) ;
#13833=CARTESIAN_POINT ( 'NONE',  ( 19.79075590726361966, -8.422956900484598108, -78.26370100276550090 ) ) ;
#13834=VERTEX_POINT ( 'NONE', #18136 ) ;
#13837=DIRECTION ( 'NONE',  ( 1.000000000000000000, 0.000000000000000000, 0.000000000000000000 ) ) ;
#13838=CARTESIAN_POINT ( 'NONE',  ( 50.00000000000000000, -42.57363661491096707, -121.3828884801879155 ) ) ;
#13839=ORIENTED_EDGE ( 'NONE', *, *, #11009, .F. ) ;
#13840=CARTESIAN_POINT ( 'NONE',  ( 30.00000000000000711, -40.00000000000001421, -120.0000000000000142 ) ) ;
#13841=ORIENTED_EDGE ( 'NONE', *, *, #9043, .T. ) ;
#13843=ORIENTED_EDGE ( 'NONE', *, *, #18889, .T. ) ;
#13844=CARTESIAN_POINT ( 'NONE',  ( 30.84782268423197849, -110.7785652318826237, 73.91276197030045125 ) ) ;
#13845=DIRECTION ( 'NONE',  ( 0.000000000000000000, 0.000000000000000000, -1.000000000000000000 ) ) ;
#13850=VERTEX_POINT ( 'NONE', #10083 ) ;
#13853=CARTESIAN_POINT ( 'NONE',  ( 50.00000000000000000, -151.4095880458873467, 44.60680010464249534 ) ) ;
#13856=DIRECTION ( 'NONE',  ( -1.000000000000000000, 0.000000000000000000, 0.000000000000000000 ) ) ;
#13860=CARTESIAN_POINT ( 'NONE',  ( 22.70866746290765903, -3.649167310370807105, -90.00000000000000000 ) ) ;
#13864=EDGE_CURVE ( 'NONE', #2489, #8874, #9318, .T. ) ;
#13865=ORIENTED_EDGE ( 'NONE', *, *, #5772, .F. ) ;
#13867=CARTESIAN_POINT ( 'NONE',  ( 30.00000000000000000, -105.0000000000000000, -90.00000000000001421 ) ) ;
#13869=FACE_OUTER_BOUND ( 'NONE', #12140, .T. ) ;
#13875=UNCERTAINTY_MEASURE_WITH_UNIT (LENGTH_MEASURE( 1.000000000000000082E-05 ), #2142, 'distance_accuracy_value', 'NONE');
#13882=EDGE_CURVE ( 'NONE', #1850, #16461, #8551, .T. ) ;
#13890=CARTESIAN_POINT ( 'NONE',  ( 30.62964503024144491, -40.90928292143731682, -71.38288848018790134 ) ) ;
#13896=CARTESIAN_POINT ( 'NONE',  ( 24.99999999999999645, -85.00000000000000000, -1.040949779275250179E-14 ) ) ;
#13911=ORIENTED_EDGE ( 'NONE', *, *, #17082, .F. ) ;
#13913=CARTESIAN_POINT ( 'NONE',  ( 16.80529800326409173, -13.48305675317432595, 74.69048503828152263 ) ) ;
#13922=ORIENTED_EDGE ( 'NONE', *, *, #6727, .F. ) ;
#13923=CARTESIAN_POINT ( 'NONE',  ( 40.00000000000000711, -122.3205080756887639, 80.28096411455982206 ) ) ;
#13927=DIRECTION ( 'NONE',  ( 1.000000000000000000, 0.000000000000000000, 0.000000000000000000 ) ) ;
#13933=VECTOR ( 'NONE', #12198, 1000.000000000000000 ) ;
#13934=CARTESIAN_POINT ( 'NONE',  ( 12.05832282520466947, -17.81513111787450043, -72.26823280878556943 ) ) ;
#13936=ORIENTED_EDGE ( 'NONE', *, *, #12570, .F. ) ;
#13938=DIRECTION ( 'NONE',  ( 0.000000000000000000, 0.000000000000000000, -1.000000000000000000 ) ) ;
#13940=AXIS2_PLACEMENT_3D ( 'NONE', #4359, #10824, #2766 ) ;
#13944=ORIENTED_EDGE ( 'NONE', *, *, #12855, .F. ) ;
#13945=CARTESIAN_POINT ( 'NONE',  ( -25.00000000000000000, -30.00000000000000711, 58.09475019311124555 ) ) ;
#13946=VECTOR ( 'NONE', #831, 1000.000000000000000 ) ;
#13950=EDGE_CURVE ( 'NONE', #5238, #5869, #10609, .T. ) ;
#13956=ORIENTED_EDGE ( 'NONE', *, *, #410, .F. ) ;
#13960=CARTESIAN_POINT ( 'NONE',  ( -19.83201477098864274, -8.377285018628274571, 84.88081099966895238 ) ) ;
#13967=ORIENTED_EDGE ( 'NONE', *, *, #1996, .T. ) ;
#13969=CARTESIAN_POINT ( 'NONE',  ( 18.48989557468869549, -13.69507619692709710, -80.56043633723008668 ) ) ;
#13970=VECTOR ( 'NONE', #18971, 1000.000000000000000 ) ;
#13971=CARTESIAN_POINT ( 'NONE',  ( 24.74873734152916072, 24.74873734152916072, -120.0000000000000142 ) ) ;
#13976=FACE_OUTER_BOUND ( 'NONE', #7742, .T. ) ;
#13978=ADVANCED_FACE ( 'NONE', ( #11869, #18339 ), #2554, .F. ) ;
#13994=DIRECTION ( 'NONE',  ( 0.000000000000000000, 0.000000000000000000, 1.000000000000000000 ) ) ;
#13995=CYLINDRICAL_SURFACE ( 'NONE', #13447, 11.49999999999999645 ) ;
#13999=VECTOR ( 'NONE', #7314, 1000.000000000000000 ) ;
#14001=VERTEX_POINT ( 'NONE', #20130 ) ;
#14008=VECTOR ( 'NONE', #6802, 1000.000000000000000 ) ;
#14018=FACE_OUTER_BOUND ( 'NONE', #11220, .T. ) ;
#14022=ORIENTED_EDGE ( 'NONE', *, *, #8676, .F. ) ;
#14027=LINE ( 'NONE', #18902, #18781 ) ;
#14043=VECTOR ( 'NONE', #14, 1000.000000000000000 ) ;
#14044=CARTESIAN_POINT ( 'NONE',  ( 50.00000000000000000, -97.49621075554985339, -111.6458212409894486 ) ) ;
#14047=EDGE_CURVE ( 'NONE', #9722, #16972, #1926, .T. ) ;
#14060=PLANE ( 'NONE',  #9542 ) ;
#14061=EDGE_LOOP ( 'NONE', ( #9855, #8106, #14070, #15064, #2995, #18993 ) ) ;
#14070=ORIENTED_EDGE ( 'NONE', *, *, #6011, .T. ) ;
#14077=CIRCLE ( 'NONE', #16767, 80.00000000000000000 ) ;
#14079=DIRECTION ( 'NONE',  ( 0.000000000000000000, 0.000000000000000000, -1.000000000000000000 ) ) ;
#14083=CARTESIAN_POINT ( 'NONE',  ( -8.500000000000000000, 1.040949779275250140E-15, 81.99999999999998579 ) ) ;
#14085=ORIENTED_EDGE ( 'NONE', *, *, #9206, .F. ) ;
#14086=DIRECTION ( 'NONE',  ( 0.000000000000000000, 0.000000000000000000, 1.000000000000000000 ) ) ;
#14087=PLANE ( 'NONE',  #1078 ) ;
#14088=CARTESIAN_POINT ( 'NONE',  ( -24.99999999999999289, 31.35083268962919689, -84.99999999999998579 ) ) ;
#14099=CARTESIAN_POINT ( 'NONE',  ( 24.99999999999999645, -99.99999999999998579, 52.00000000000000000 ) ) ;
#14105=DIRECTION ( 'NONE',  ( 1.000000000000000000, -0.000000000000000000, -0.000000000000000000 ) ) ;
#14109=CARTESIAN_POINT ( 'NONE',  ( 38.55055242192437959, -18.08242209349172924, -77.76562703327597603 ) ) ;
#14114=CARTESIAN_POINT ( 'NONE',  ( 38.52966308413987662, -121.3895969659597398, -79.56471955312994737 ) ) ;
#14122=VECTOR ( 'NONE', #1505, 1000.000000000000000 ) ;
#14124=CARTESIAN_POINT ( 'NONE',  ( -24.99999999999999289, -127.3290820621008379, 85.00000000000000000 ) ) ;
#14131=DIRECTION ( 'NONE',  ( -1.000000000000000000, 1.734723475976807094E-16, 0.000000000000000000 ) ) ;
#14133=DIRECTION ( 'NONE',  ( -1.000000000000000000, 0.000000000000000000, 0.000000000000000000 ) ) ;
#14135=CARTESIAN_POINT ( 'NONE',  ( 30.00000000000000000, -151.4095880458873467, 44.60680010464249534 ) ) ;
#14143=CIRCLE ( 'NONE', #11085, 3.199999999999994404 ) ;
#14147=CARTESIAN_POINT ( 'NONE',  ( -24.99999999999999289, -148.4917293642369884, -48.67032260359990659 ) ) ;
#14156=DIRECTION ( 'NONE',  ( 1.000000000000000000, -0.000000000000000000, -0.000000000000000000 ) ) ;
#14169=ORIENTED_EDGE ( 'NONE', *, *, #3910, .T. ) ;
#14171=EDGE_CURVE ( 'NONE', #20704, #2621, #11021, .T. ) ;
#14172=CARTESIAN_POINT ( 'NONE',  ( 34.75286706568503803, -117.9715115446175275, 77.27478996839415970 ) ) ;
#14183=DIRECTION ( 'NONE',  ( 0.000000000000000000, 0.000000000000000000, -1.000000000000000000 ) ) ;
#14185=ADVANCED_FACE ( 'NONE', ( #7838 ), #14320, .T. ) ;
#14187=DIRECTION ( 'NONE',  ( 0.000000000000000000, 0.000000000000000000, -1.000000000000000000 ) ) ;
#14189=VERTEX_POINT ( 'NONE', #4975 ) ;
#14193=EDGE_CURVE ( 'NONE', #2104, #15865, #18064, .T. ) ;
#14196=FACE_BOUND ( 'NONE', #5558, .T. ) ;
#14198=DIRECTION ( 'NONE',  ( 0.000000000000000000, 0.000000000000000000, -1.000000000000000000 ) ) ;
#14202=VERTEX_POINT ( 'NONE', #19591 ) ;
#14210=CARTESIAN_POINT ( 'NONE',  ( 0.000000000000000000, 0.000000000000000000, -81.99999999999998579 ) ) ;
#14211=VERTEX_POINT ( 'NONE', #17705 ) ;
#14213=CARTESIAN_POINT ( 'NONE',  ( 30.00000000000000711, -30.00000000000001421, -120.0000000000000142 ) ) ;
#14216=CARTESIAN_POINT ( 'NONE',  ( 35.30716229119248339, -118.5958850092678460, -77.65589229240622160 ) ) ;
#14219=ADVANCED_FACE ( 'NONE', ( #14425 ), #6756, .F. ) ;
#14223=CARTESIAN_POINT ( 'NONE',  ( 8.500000000000000000, 0.000000000000000000, 90.00000000000000000 ) ) ;
#14225=CARTESIAN_POINT ( 'NONE',  ( 30.00000000000000000, -39.99999999999999289, 52.00000000000000000 ) ) ;
#14228=ORIENTED_EDGE ( 'NONE', *, *, #20198, .T. ) ;
#14232=CARTESIAN_POINT ( 'NONE',  ( -11.50000000000000000, 1.408343819019456176E-15, 68.00000000000000000 ) ) ;
#14238=VERTEX_POINT ( 'NONE', #9650 ) ;
#14242=CYLINDRICAL_SURFACE ( 'NONE', #17076, 35.00000000000000000 ) ;
#14244=DIRECTION ( 'NONE',  ( 1.000000000000000000, 0.000000000000000000, 0.000000000000000000 ) ) ;
#14250=EDGE_CURVE ( 'NONE', #20337, #14343, #17385, .T. ) ;
#14253=EDGE_CURVE ( 'NONE', #11718, #20455, #1482, .T. ) ;
#14257=CARTESIAN_POINT ( 'NONE',  ( 30.00000000000000000, -122.0000000000000000, -2.100000000000004086 ) ) ;
#14263=VERTEX_POINT ( 'NONE', #8251 ) ;
#14266=PLANE ( 'NONE',  #7703 ) ;
#14274=CARTESIAN_POINT ( 'NONE',  ( 7.653695106945543891, -20.10381028312655971, 76.71523333892115204 ) ) ;
#14277=EDGE_CURVE ( 'NONE', #12734, #10607, #1140, .T. ) ;
#14280=ORIENTED_EDGE ( 'NONE', *, *, #11299, .F. ) ;
#14287=CYLINDRICAL_SURFACE ( 'NONE', #1790, 23.00000000000000000 ) ;
#14290=ORIENTED_EDGE ( 'NONE', *, *, #1222, .F. ) ;
#14293=AXIS2_PLACEMENT_3D ( 'NONE', #10738, #12529, #13812 ) ;
#14295=CARTESIAN_POINT ( 'NONE',  ( 30.00000000000000000, -164.9999999999999716, -50.00000000000002132 ) ) ;
#14301=EDGE_CURVE ( 'NONE', #12434, #18682, #11108, .T. ) ;
#14304=CARTESIAN_POINT ( 'NONE',  ( -27.96694501150314593, -24.74873734152930993, -130.0000000000000000 ) ) ;
#14311=AXIS2_PLACEMENT_3D ( 'NONE', #18302, #10463, #508 ) ;
#14318=EDGE_LOOP ( 'NONE', ( #8843, #5479, #3986, #16382 ) ) ;
#14320=PLANE ( 'NONE',  #20756 ) ;
#14323=ORIENTED_EDGE ( 'NONE', *, *, #2649, .T. ) ;
#14324=CARTESIAN_POINT ( 'NONE',  ( 50.00000000000000000, 31.35083268962916137, 50.63110039191614220 ) ) ;
#14333=CARTESIAN_POINT ( 'NONE',  ( -24.99999999999999289, -159.9999999999999716, 85.00000000000000000 ) ) ;
#14334=VECTOR ( 'NONE', #7454, 1000.000000000000000 ) ;
#14335=DIRECTION ( 'NONE',  ( -0.000000000000000000, -0.000000000000000000, 1.000000000000000000 ) ) ;
#14341=DIRECTION ( 'NONE',  ( 0.000000000000000000, 0.000000000000000000, 1.000000000000000000 ) ) ;
#14343=VERTEX_POINT ( 'NONE', #14508 ) ;
#14348=FACE_OUTER_BOUND ( 'NONE', #3368, .T. ) ;
#14356=DIRECTION ( 'NONE',  ( 0.000000000000000000, 0.000000000000000000, 1.000000000000000000 ) ) ;
#14358=CYLINDRICAL_SURFACE ( 'NONE', #19089, 39.99999999999999289 ) ;
#14363=EDGE_LOOP ( 'NONE', ( #991, #10099, #6586, #10988 ) ) ;
#14364=CARTESIAN_POINT ( 'NONE',  ( 19.74873734152915716, 24.74873734152916072, -120.0000000000000142 ) ) ;
#14367=DIRECTION ( 'NONE',  ( 0.000000000000000000, 0.000000000000000000, -1.000000000000000000 ) ) ;
#14388=ORIENTED_EDGE ( 'NONE', *, *, #5358, .T. ) ;
#14392=ORIENTED_EDGE ( 'NONE', *, *, #7956, .F. ) ;
#14393=DIRECTION ( 'NONE',  ( -0.000000000000000000, -0.000000000000000000, 1.000000000000000000 ) ) ;
#14396=ORIENTED_EDGE ( 'NONE', *, *, #210, .F. ) ;
#14397=CARTESIAN_POINT ( 'NONE',  ( -10.27973195343232149, -20.58856569599344510, -76.47391966369774252 ) ) ;
#14409=LINE ( 'NONE', #6339, #7911 ) ;
#14411=EDGE_LOOP ( 'NONE', ( #4408, #8061 ) ) ;
#14412=CARTESIAN_POINT ( 'NONE',  ( -21.45900938229203447, -1.326995226329880762, -84.99999999999998579 ) ) ;
#14420=EDGE_LOOP ( 'NONE', ( #1895, #11714 ) ) ;
#14422=DIRECTION ( 'NONE',  ( 0.000000000000000000, 0.000000000000000000, 1.000000000000000000 ) ) ;
#14424=CARTESIAN_POINT ( 'NONE',  ( 24.99999999999999645, -85.00000000000000000, -1.040949779275250179E-14 ) ) ;
#14425=FACE_OUTER_BOUND ( 'NONE', #12298, .T. ) ;
#14426=EDGE_LOOP ( 'NONE', ( #4291, #18999, #10721, #11605 ) ) ;
#14427=ORIENTED_EDGE ( 'NONE', *, *, #17922, .F. ) ;
#14428=CARTESIAN_POINT ( 'NONE',  ( 50.00000000000000000, -42.57363661491096707, -121.3828884801879155 ) ) ;
#14429=EDGE_CURVE ( 'NONE', #16465, #13160, #17113, .T. ) ;
#14433=AXIS2_PLACEMENT_3D ( 'NONE', #19605, #5081, #12849 ) ;
#14463=AXIS2_PLACEMENT_3D ( 'NONE', #9950, #205, #16615 ) ;
#14464=VECTOR ( 'NONE', #20766, 1000.000000000000000 ) ;
#14466=ORIENTED_EDGE ( 'NONE', *, *, #13864, .F. ) ;
#14478=AXIS2_PLACEMENT_3D ( 'NONE', #3800, #10284, #10390 ) ;
#14483=CIRCLE ( 'NONE', #3943, 21.50000000000000000 ) ;
#14484=ORIENTED_EDGE ( 'NONE', *, *, #1646, .F. ) ;
#14485=AXIS2_PLACEMENT_3D ( 'NONE', #8020, #15566, #14500 ) ;
#14486=CARTESIAN_POINT ( 'NONE',  ( 39.99999999999997158, -122.3205080756887497, -80.28096411455980785 ) ) ;
#14487=CARTESIAN_POINT ( 'NONE',  ( -26.35784117651625280, 26.35784117651607872, -120.0000000000000142 ) ) ;
#14493=EDGE_CURVE ( 'NONE', #19457, #17375, #4387, .T. ) ;
#14497=CARTESIAN_POINT ( 'NONE',  ( -24.99999999999999289, -42.57363661491096707, 121.3828884801879155 ) ) ;
#14498=AXIS2_PLACEMENT_3D ( 'NONE', #19878, #15006, #6276 ) ;
#14499=DIRECTION ( 'NONE',  ( 1.000000000000000000, 0.000000000000000000, 0.000000000000000000 ) ) ;
#14500=DIRECTION ( 'NONE',  ( -1.000000000000000000, 0.000000000000000000, 0.000000000000000000 ) ) ;
#14505=EDGE_LOOP ( 'NONE', ( #343, #13657 ) ) ;
#14506=CARTESIAN_POINT ( 'NONE',  ( -13.44994733502084294, -18.67183681267612982, -77.46342352758064465 ) ) ;
#14508=CARTESIAN_POINT ( 'NONE',  ( 29.74873734152916782, 24.74873734152916072, -130.0000000000000000 ) ) ;
#14518=DIRECTION ( 'NONE',  ( -0.000000000000000000, -0.000000000000000000, 1.000000000000000000 ) ) ;
#14525=CARTESIAN_POINT ( 'NONE',  ( 30.00000000000000000, -39.99999999999999289, -52.00000000000000000 ) ) ;
#14529=VERTEX_POINT ( 'NONE', #20698 ) ;
#14530=EDGE_CURVE ( 'NONE', #15865, #8953, #6219, .T. ) ;
#14535=FACE_OUTER_BOUND ( 'NONE', #16585, .T. ) ;
#14539=FACE_OUTER_BOUND ( 'NONE', #10335, .T. ) ;
#14543=ORIENTED_EDGE ( 'NONE', *, *, #15687, .T. ) ;
#14548=LINE ( 'NONE', #1817, #5901 ) ;
#14553=CARTESIAN_POINT ( 'NONE',  ( 37.43953707193390557, -20.06695501706099094, 76.69796010862685876 ) ) ;
#14577=VERTEX_POINT ( 'NONE', #3516 ) ;
#14584=CARTESIAN_POINT ( 'NONE',  ( 40.00000000000000711, 29.99999999999999289, -130.0000000000000000 ) ) ;
#14593=CIRCLE ( 'NONE', #4767, 10.00000000000000178 ) ;
#14595=CYLINDRICAL_SURFACE ( 'NONE', #4134, 8.999999999999994671 ) ;
#14596=DIRECTION ( 'NONE',  ( 1.000000000000000000, 0.000000000000000000, 0.000000000000000000 ) ) ;
#14598=EDGE_CURVE ( 'NONE', #4487, #14705, #4181, .T. ) ;
#14611=B_SPLINE_CURVE_WITH_KNOTS ( 'NONE', 3,
 ( #20053, #8819, #2164, #7344 ),
 .UNSPECIFIED., .F., .F.,
 ( 4, 4 ),
 ( 6.938893903907228378E-18, 0.007425583459339141733 ),
 .UNSPECIFIED. ) ;
#14612=EDGE_LOOP ( 'NONE', ( #19759, #16256, #19540, #3707 ) ) ;
#14620=DIRECTION ( 'NONE',  ( 0.000000000000000000, 0.000000000000000000, -1.000000000000000000 ) ) ;
#14621=DIRECTION ( 'NONE',  ( 0.000000000000000000, 0.000000000000000000, -1.000000000000000000 ) ) ;
#14623=ORIENTED_EDGE ( 'NONE', *, *, #4138, .F. ) ;
#14624=EDGE_LOOP ( 'NONE', ( #10979, #8753, #3279, #10318, #1917, #13493 ) ) ;
#14626=DIRECTION ( 'NONE',  ( 0.000000000000000000, 0.000000000000000000, -1.000000000000000000 ) ) ;
#14628=ADVANCED_FACE ( 'NONE', ( #14867 ), #13074, .F. ) ;
#14632=AXIS2_PLACEMENT_3D ( 'NONE', #18877, #2753, #9220 ) ;
#14643=CARTESIAN_POINT ( 'NONE',  ( 50.00000000000000000, 31.35083268962916137, -50.63110039191615641 ) ) ;
#14647=CIRCLE ( 'NONE', #16679, 11.49999999999999645 ) ;
#14652=DIRECTION ( 'NONE',  ( 0.000000000000000000, 0.000000000000000000, 1.000000000000000000 ) ) ;
#14658=EDGE_CURVE ( 'NONE', #17751, #1745, #17947, .T. ) ;
#14660=EDGE_CURVE ( 'NONE', #20532, #12434, #1649, .T. ) ;
#14661=AXIS2_PLACEMENT_3D ( 'NONE', #16063, #4401, #1556 ) ;
#14667=VERTEX_POINT ( 'NONE', #19428 ) ;
#14669=DIRECTION ( 'NONE',  ( 0.000000000000000000, 0.000000000000000000, -1.000000000000000000 ) ) ;
#14671=DIRECTION ( 'NONE',  ( 0.000000000000000000, 1.040834085586084454E-15, -1.000000000000000000 ) ) ;
#14682=ADVANCED_FACE ( 'NONE', ( #2247 ), #2350, .T. ) ;
#14683=CARTESIAN_POINT ( 'NONE',  ( 40.00000000000000711, -122.3205080756887781, -90.00000000000001421 ) ) ;
#14690=AXIS2_PLACEMENT_3D ( 'NONE', #4602, #15934, #1431 ) ;
#14696=ORIENTED_EDGE ( 'NONE', *, *, #3673, .T. ) ;
#14701=EDGE_CURVE ( 'NONE', #17868, #14994, #11969, .T. ) ;
#14703=CARTESIAN_POINT ( 'NONE',  ( 29.99999999999966249, -160.0000000000000000, 53.99496054166689163 ) ) ;
#14705=VERTEX_POINT ( 'NONE', #16552 ) ;
#14707=CARTESIAN_POINT ( 'NONE',  ( 29.99999999999965183, -159.9999999999999716, 53.99496054166689873 ) ) ;
#14714=FACE_BOUND ( 'NONE', #878, .T. ) ;
#14717=DIRECTION ( 'NONE',  ( 0.000000000000000000, 0.000000000000000000, -1.000000000000000000 ) ) ;
#14720=DIRECTION ( 'NONE',  ( -0.000000000000000000, -0.000000000000000000, 1.000000000000000000 ) ) ;
#14723=CARTESIAN_POINT ( 'NONE',  ( -11.50000000000000000, 1.408343819019456176E-15, 81.99999999999998579 ) ) ;
#14728=VERTEX_POINT ( 'NONE', #15273 ) ;
#14734=CARTESIAN_POINT ( 'NONE',  ( 30.00000000000000355, -139.6410161513775563, -90.00000000000001421 ) ) ;
#14744=DIRECTION ( 'NONE',  ( -0.000000000000000000, -0.000000000000000000, 1.000000000000000000 ) ) ;
#14747=VERTEX_POINT ( 'NONE', #8709 ) ;
#14749=CARTESIAN_POINT ( 'NONE',  ( 35.80519692130376797, -23.36569907514590838, 75.18387685020788069 ) ) ;
#14751=ORIENTED_EDGE ( 'NONE', *, *, #16207, .T. ) ;
#14755=CARTESIAN_POINT ( 'NONE',  ( 30.00000000000000000, -122.0000000000000000, 2.099999999999991207 ) ) ;
#14766=ORIENTED_EDGE ( 'NONE', *, *, #12468, .T. ) ;
#14768=ORIENTED_EDGE ( 'NONE', *, *, #11943, .T. ) ;
#14773=CARTESIAN_POINT ( 'NONE',  ( 50.00100000000000477, -85.00000000000000000, -1.040949779275250179E-14 ) ) ;
#14775=CARTESIAN_POINT ( 'NONE',  ( -30.00000000000000000, -85.00000000000000000, -1.040949779275250179E-14 ) ) ;
#14781=DIRECTION ( 'NONE',  ( -1.000000000000000000, -0.000000000000000000, -0.000000000000000000 ) ) ;
#14784=DIRECTION ( 'NONE',  ( -1.000000000000000000, 0.000000000000000000, 0.000000000000000000 ) ) ;
#14789=DIRECTION ( 'NONE',  ( 0.000000000000000000, 0.000000000000000000, -1.000000000000000000 ) ) ;
#14796=DIRECTION ( 'NONE',  ( -1.000000000000000000, 0.000000000000000000, 0.000000000000000000 ) ) ;
#14802=EDGE_CURVE ( 'NONE', #8802, #13140, #14972, .T. ) ;
#14816=ORIENTED_EDGE ( 'NONE', *, *, #5658, .T. ) ;
#14828=CARTESIAN_POINT ( 'NONE',  ( 30.11504063214072602, -46.04687138839951643, 66.48368087637908275 ) ) ;
#14833=CARTESIAN_POINT ( 'NONE',  ( 24.74873734152916072, 24.74873734152916072, -130.0000000000000000 ) ) ;
#14834=ORIENTED_EDGE ( 'NONE', *, *, #8419, .T. ) ;
#14838=LINE ( 'NONE', #14935, #4479 ) ;
#14839=DIRECTION ( 'NONE',  ( 0.000000000000000000, 0.000000000000000000, -1.000000000000000000 ) ) ;
#14843=LINE ( 'NONE', #13048, #4022 ) ;
#14844=CARTESIAN_POINT ( 'NONE',  ( -30.00000000000000000, -85.00000000000000000, 14.49999999999998579 ) ) ;
#14848=CARTESIAN_POINT ( 'NONE',  ( -30.00000000000000000, -3.649167310370820871, 90.00000000000000000 ) ) ;
#14851=VERTEX_POINT ( 'NONE', #15075 ) ;
#14852=CARTESIAN_POINT ( 'NONE',  ( 30.00000000000000000, -39.99999999999999289, -52.00000000000000000 ) ) ;
#14853=CARTESIAN_POINT ( 'NONE',  ( 31.92289614601317282, -34.44341132653233473, -66.98101497439323282 ) ) ;
#14854=EDGE_LOOP ( 'NONE', ( #1209, #3314, #1139, #7164 ) ) ;
#14855=ORIENTED_EDGE ( 'NONE', *, *, #6286, .F. ) ;
#14856=CARTESIAN_POINT ( 'NONE',  ( 24.99999999999999645, -30.00000000000000711, -1.040949779275250179E-14 ) ) ;
#14862=PLANE ( 'NONE',  #13331 ) ;
#14867=FACE_OUTER_BOUND ( 'NONE', #3995, .T. ) ;
#14876=DIRECTION ( 'NONE',  ( 0.000000000000000000, 0.000000000000000000, -1.000000000000000000 ) ) ;
#14878=EDGE_LOOP ( 'NONE', ( #8082, #16331, #10540, #19876, #18281, #10340 ) ) ;
#14879=EDGE_CURVE ( 'NONE', #12782, #13834, #10977, .T. ) ;
#14886=EDGE_CURVE ( 'NONE', #10522, #231, #16990, .T. ) ;
#14887=VERTEX_POINT ( 'NONE', #10432 ) ;
#14888=CARTESIAN_POINT ( 'NONE',  ( 50.00000000000000000, -97.49621075554985339, 111.6458212409894486 ) ) ;
#14895=DIRECTION ( 'NONE',  ( 0.000000000000000000, 0.000000000000000000, 1.000000000000000000 ) ) ;
#14899=ORIENTED_EDGE ( 'NONE', *, *, #4912, .T. ) ;
#14914=ORIENTED_EDGE ( 'NONE', *, *, #2211, .F. ) ;
#14927=PLANE ( 'NONE',  #19672 ) ;
#14932=CARTESIAN_POINT ( 'NONE',  ( 47.05877748208924061, -6.233954241158976117, -80.06349855976149854 ) ) ;
#14933=EDGE_CURVE ( 'NONE', #14851, #1850, #14611, .T. ) ;
#14934=CARTESIAN_POINT ( 'NONE',  ( -11.50000000000000000, 1.408343819019456176E-15, 68.00000000000000000 ) ) ;
#14935=CARTESIAN_POINT ( 'NONE',  ( 10.00000000000000178, -148.4917293642369884, -48.67032260359990659 ) ) ;
#14939=UNCERTAINTY_MEASURE_WITH_UNIT (LENGTH_MEASURE( 1.000000000000000082E-05 ), #5009, 'distance_accuracy_value', 'NONE');
#14941=CARTESIAN_POINT ( 'NONE',  ( 30.00000000000000000, -148.4917293642369600, 48.67032260359987816 ) ) ;
#14945=CARTESIAN_POINT ( 'NONE',  ( 50.00000000000000000, 36.35083268962920044, -90.00000000000000000 ) ) ;
#14954=DIRECTION ( 'NONE',  ( 0.000000000000000000, 0.000000000000000000, 1.000000000000000000 ) ) ;
#14955=EDGE_LOOP ( 'NONE', ( #3463, #12980, #927, #11508, #9692, #13513, #7482, #10628, #4900, #19610, #9042, #17568 ) ) ;
#14963=LINE ( 'NONE', #8281, #4210 ) ;
#14970=( NAMED_UNIT ( * ) PLANE_ANGLE_UNIT ( ) SI_UNIT ( $, .RADIAN. ) );
#14972=LINE ( 'NONE', #560, #16374 ) ;
#14976=ORIENTED_EDGE ( 'NONE', *, *, #13882, .T. ) ;
#14978=CARTESIAN_POINT ( 'NONE',  ( -19.81419003091921383, -8.351337688303456019, 78.32518794914261662 ) ) ;
#14981=LINE ( 'NONE', #16772, #5868 ) ;
#14983=DIRECTION ( 'NONE',  ( 0.000000000000000000, 0.000000000000000000, -1.000000000000000000 ) ) ;
#14987=DIRECTION ( 'NONE',  ( 0.000000000000000000, 0.000000000000000000, -1.000000000000000000 ) ) ;
#14989=DIRECTION ( 'NONE',  ( -1.000000000000000000, 0.000000000000000000, 0.000000000000000000 ) ) ;
#14992=AXIS2_PLACEMENT_3D ( 'NONE', #14487, #1245, #7698 ) ;
#14994=VERTEX_POINT ( 'NONE', #12337 ) ;
#15004=AXIS2_PLACEMENT_3D ( 'NONE', #6256, #12306, #9334 ) ;
#15006=DIRECTION ( 'NONE',  ( 0.000000000000000000, -1.000000000000000000, 0.000000000000000000 ) ) ;
#15027=ORIENTED_EDGE ( 'NONE', *, *, #3343, .T. ) ;
#15028=DIRECTION ( 'NONE',  ( 1.000000000000000000, 0.000000000000000000, 0.000000000000000000 ) ) ;
#15029=CARTESIAN_POINT ( 'NONE',  ( 39.99999999999997158, -122.3205080756887497, -80.28096411455980785 ) ) ;
#15031=VERTEX_POINT ( 'NONE', #14147 ) ;
#15046=DIRECTION ( 'NONE',  ( 0.000000000000000000, 0.000000000000000000, -1.000000000000000000 ) ) ;
#15049=DIRECTION ( 'NONE',  ( 0.000000000000000000, 0.000000000000000000, -1.000000000000000000 ) ) ;
#15051=EDGE_CURVE ( 'NONE', #19712, #6167, #5225, .T. ) ;
#15052=AXIS2_PLACEMENT_3D ( 'NONE', #1916, #16133, #3393 ) ;
#15054=DIRECTION ( 'NONE',  ( 0.000000000000000000, 0.000000000000000000, -1.000000000000000000 ) ) ;
#15056=FACE_BOUND ( 'NONE', #12282, .T. ) ;
#15061=CARTESIAN_POINT ( 'NONE',  ( 24.99999999999999645, -39.99999999999999289, 49.89999999999999858 ) ) ;
#15064=ORIENTED_EDGE ( 'NONE', *, *, #824, .F. ) ;
#15067=CARTESIAN_POINT ( 'NONE',  ( 50.00000000000000000, -97.49621075554985339, 111.6458212409894486 ) ) ;
#15073=DIRECTION ( 'NONE',  ( 0.000000000000000000, 0.000000000000000000, -1.000000000000000000 ) ) ;
#15075=CARTESIAN_POINT ( 'NONE',  ( 30.00000000000000000, -50.00000000000000000, -66.88656633939928042 ) ) ;
#15076=ADVANCED_FACE ( 'NONE', ( #7664 ), #14242, .F. ) ;
#15079=EDGE_LOOP ( 'NONE', ( #4311, #6662, #11367, #2743 ) ) ;
#15081=CARTESIAN_POINT ( 'NONE',  ( 2.601994274788632211, -21.34541601844983916, 70.64469287327099778 ) ) ;
#15084=ORIENTED_EDGE ( 'NONE', *, *, #16101, .F. ) ;
#15086=LINE ( 'NONE', #2465, #9505 ) ;
#15089=ORIENTED_EDGE ( 'NONE', *, *, #16958, .T. ) ;
#15097=ORIENTED_EDGE ( 'NONE', *, *, #5089, .F. ) ;
#15103=ORIENTED_EDGE ( 'NONE', *, *, #8065, .F. ) ;
#15106=CARTESIAN_POINT ( 'NONE',  ( 10.00000000000000178, -164.9999999999999716, -70.00000000000000000 ) ) ;
#15107=DIRECTION ( 'NONE',  ( -1.000000000000000000, 0.000000000000000000, 0.000000000000000000 ) ) ;
#15108=ORIENTED_EDGE ( 'NONE', *, *, #4679, .F. ) ;
#15110=ORIENTED_EDGE ( 'NONE', *, *, #6598, .T. ) ;
#15112=AXIS2_PLACEMENT_3D ( 'NONE', #19180, #9432, #13994 ) ;
#15118=AXIS2_PLACEMENT_3D ( 'NONE', #2891, #20900, #1102 ) ;
#15126=AXIS2_PLACEMENT_3D ( 'NONE', #2466, #10024, #9145 ) ;
#15129=ORIENTED_EDGE ( 'NONE', *, *, #3012, .T. ) ;
#15134=ORIENTED_EDGE ( 'NONE', *, *, #19126, .F. ) ;
#15140=CARTESIAN_POINT ( 'NONE',  ( 47.99913302141636251, -4.465704580667236634, -88.98724172780555364 ) ) ;
#15160=ORIENTED_EDGE ( 'NONE', *, *, #2081, .T. ) ;
#15162=CARTESIAN_POINT ( 'NONE',  ( 50.00000000000000000, -42.57363661491096707, 121.3828884801879155 ) ) ;
#15163=ORIENTED_EDGE ( 'NONE', *, *, #17982, .F. ) ;
#15169=( NAMED_UNIT ( * ) SI_UNIT ( $, .STERADIAN. ) SOLID_ANGLE_UNIT ( ) );
#15170=DIRECTION ( 'NONE',  ( 0.000000000000000000, 0.000000000000000000, -1.000000000000000000 ) ) ;
#15174=EDGE_CURVE ( 'NONE', #16423, #19553, #20795, .T. ) ;
#15175=LINE ( 'NONE', #10190, #5408 ) ;
#15184=CARTESIAN_POINT ( 'NONE',  ( -17.67520963998170203, -12.31071423659304109, 75.43714694428801693 ) ) ;
#15187=ORIENTED_EDGE ( 'NONE', *, *, #13240, .T. ) ;
#15195=EDGE_CURVE ( 'NONE', #13187, #7518, #9621, .T. ) ;
#15201=DIRECTION ( 'NONE',  ( -1.000000000000000000, 0.000000000000000000, 0.000000000000000000 ) ) ;
#15203=CARTESIAN_POINT ( 'NONE',  ( -16.87108763463411165, -13.40169213801852699, -74.74090047603391440 ) ) ;
#15204=ORIENTED_EDGE ( 'NONE', *, *, #2472, .F. ) ;
#15206=CYLINDRICAL_SURFACE ( 'NONE', #2923, 40.00000000000000000 ) ;
#15212=ORIENTED_EDGE ( 'NONE', *, *, #17647, .T. ) ;
#15213=DIRECTION ( 'NONE',  ( 1.000000000000000000, -0.000000000000000000, -0.000000000000000000 ) ) ;
#15216=DIRECTION ( 'NONE',  ( 1.000000000000000000, 0.000000000000000000, 0.000000000000000000 ) ) ;
#15219=ORIENTED_EDGE ( 'NONE', *, *, #4934, .F. ) ;
#15221=DIRECTION ( 'NONE',  ( 0.000000000000000000, 1.000000000000000000, -3.469446951953615175E-16 ) ) ;
#15229=STYLED_ITEM ( 'NONE', ( #8707 ), #3565 ) ;
#15230=ORIENTED_EDGE ( 'NONE', *, *, #8849, .F. ) ;
#15232=ORIENTED_EDGE ( 'NONE', *, *, #4302, .T. ) ;
#15237=CARTESIAN_POINT ( 'NONE',  ( 30.00000000000000000, -170.8299878242309546, -15.48896927112552824 ) ) ;
#15238=CIRCLE ( 'NONE', #18283, 80.00000000000000000 ) ;
#15243=CARTESIAN_POINT ( 'NONE',  ( 50.00000000000000000, 36.35083268962915781, -50.00000000000000000 ) ) ;
#15245=VECTOR ( 'NONE', #7116, 1000.000000000000000 ) ;
#15249=ORIENTED_EDGE ( 'NONE', *, *, #13003, .T. ) ;
#15255=CARTESIAN_POINT ( 'NONE',  ( -21.50000000000000000, 2.632990618166809235E-15, 68.00000000000000000 ) ) ;
#15257=CARTESIAN_POINT ( 'NONE',  ( 30.00000000000000000, -39.99999999999999289, -54.09999999999998721 ) ) ;
#15263=ORIENTED_EDGE ( 'NONE', *, *, #20300, .F. ) ;
#15265=EDGE_CURVE ( 'NONE', #13795, #8524, #14963, .T. ) ;
#15272=FACE_OUTER_BOUND ( 'NONE', #15079, .T. ) ;
#15273=CARTESIAN_POINT ( 'NONE',  ( -30.00000000000000000, -124.9999999999999858, -90.00000000000001421 ) ) ;
#15278=CARTESIAN_POINT ( 'NONE',  ( -13.88581415360056326, -16.42997871820714906, 72.99065141121243983 ) ) ;
#15282=ORIENTED_EDGE ( 'NONE', *, *, #19581, .T. ) ;
#15288=EDGE_CURVE ( 'NONE', #11798, #10778, #5010, .T. ) ;
#15291=VECTOR ( 'NONE', #16832, 1000.000000000000000 ) ;
#15295=CARTESIAN_POINT ( 'NONE',  ( -24.99999999999999289, -29.99999999999999289, -58.09475019311125976 ) ) ;
#15302=ORIENTED_EDGE ( 'NONE', *, *, #12206, .F. ) ;
#15304=CARTESIAN_POINT ( 'NONE',  ( -10.58466049171558865, -18.71773173394921486, -71.82544846116152826 ) ) ;
#15306=VERTEX_POINT ( 'NONE', #8179 ) ;
#15309=FACE_OUTER_BOUND ( 'NONE', #9688, .T. ) ;
#15311=ORIENTED_EDGE ( 'NONE', *, *, #9224, .T. ) ;
#15322=LINE ( 'NONE', #19774, #4309 ) ;
#15330=ORIENTED_EDGE ( 'NONE', *, *, #16553, .F. ) ;
#15337=VERTEX_POINT ( 'NONE', #9679 ) ;
#15340=VERTEX_POINT ( 'NONE', #8908 ) ;
#15346=AXIS2_PLACEMENT_3D ( 'NONE', #1604, #199, #13144 ) ;
#15355=CIRCLE ( 'NONE', #476, 35.00000000000000000 ) ;
#15362=AXIS2_PLACEMENT_3D ( 'NONE', #4032, #8801, #5412 ) ;
#15366=LINE ( 'NONE', #5815, #13970 ) ;
#15378=LINE ( 'NONE', #16865, #1585 ) ;
#15379=CARTESIAN_POINT ( 'NONE',  ( 21.50000000000000000, 0.000000000000000000, 68.00000000000000000 ) ) ;
#15380=EDGE_CURVE ( 'NONE', #14705, #4487, #11955, .T. ) ;
#15382=CIRCLE ( 'NONE', #3861, 2.099999999999990763 ) ;
#15385=LINE ( 'NONE', #9428, #4418 ) ;
#15386=CARTESIAN_POINT ( 'NONE',  ( 19.74873734152915716, 24.74873734152916072, -120.0000000000000142 ) ) ;
#15389=CYLINDRICAL_SURFACE ( 'NONE', #14293, 8.500000000000000000 ) ;
#15392=CARTESIAN_POINT ( 'NONE',  ( 7.417002224176399316, -20.23665979631133638, 71.11836349014902225 ) ) ;
#15398=DIRECTION ( 'NONE',  ( -1.000000000000000000, 0.000000000000000000, 0.000000000000000000 ) ) ;
#15399=DIRECTION ( 'NONE',  ( 0.000000000000000000, -0.000000000000000000, 1.000000000000000000 ) ) ;
#15402=DIRECTION ( 'NONE',  ( -0.000000000000000000, -1.000000000000000000, -0.000000000000000000 ) ) ;
#15409=ORIENTED_EDGE ( 'NONE', *, *, #1646, .T. ) ;
#15410=CARTESIAN_POINT ( 'NONE',  ( 50.00000000000000000, 36.35083268962917202, 90.00000000000000000 ) ) ;
#15412=ORIENTED_EDGE ( 'NONE', *, *, #3404, .T. ) ;
#15413=DIRECTION ( 'NONE',  ( -1.000000000000000000, 5.334274688628681815E-15, 0.000000000000000000 ) ) ;
#15415=VERTEX_POINT ( 'NONE', #13483 ) ;
#15418=CARTESIAN_POINT ( 'NONE',  ( 30.00000000000000711, 29.99999999999998579, -130.0000000000000000 ) ) ;
#15423=CARTESIAN_POINT ( 'NONE',  ( 28.13963350654227824, -26.35784117651622793, -120.0000000000000142 ) ) ;
#15437=ADVANCED_FACE ( 'NONE', ( #7098 ), #751, .F. ) ;
#15440=CARTESIAN_POINT ( 'NONE',  ( 50.00000000000000000, 36.35083268962915781, 50.00000000000000000 ) ) ;
#15441=AXIS2_PLACEMENT_3D ( 'NONE', #12234, #13519, #18709 ) ;
#15449=DIRECTION ( 'NONE',  ( 0.000000000000000000, -3.469446951953615175E-16, -1.000000000000000000 ) ) ;
#15456=CARTESIAN_POINT ( 'NONE',  ( 30.00000000000000000, -164.9999999999999716, -50.00000000000002842 ) ) ;
#15459=VECTOR ( 'NONE', #2868, 1000.000000000000000 ) ;
#15463=EDGE_CURVE ( 'NONE', #10607, #15704, #8595, .T. ) ;
#15466=DIRECTION ( 'NONE',  ( -1.000000000000000000, 0.000000000000000000, 0.000000000000000000 ) ) ;
#15471=ADVANCED_FACE ( 'NONE', ( #4128 ), #2560, .F. ) ;
#15473=LINE ( 'NONE', #7504, #1623 ) ;
#15481=ORIENTED_EDGE ( 'NONE', *, *, #12542, .T. ) ;
#15487=PLANE ( 'NONE',  #12296 ) ;
#15497=ORIENTED_EDGE ( 'NONE', *, *, #7995, .T. ) ;
#15503=LINE ( 'NONE', #10523, #15245 ) ;
#15506=ADVANCED_FACE ( 'NONE', ( #2342, #9024 ), #15487, .T. ) ;
#15507=ORIENTED_EDGE ( 'NONE', *, *, #16603, .F. ) ;
#15509=CARTESIAN_POINT ( 'NONE',  ( 45.22159793441011999, -8.673994507468384185, 84.62946326583127643 ) ) ;
#15516=CARTESIAN_POINT ( 'NONE',  ( 5.982253535725074123, -20.70709046307243995, -70.91533586927070587 ) ) ;
#15520=CARTESIAN_POINT ( 'NONE',  ( 93.70999227554992217, -50.00000000000000000, -90.00000000000001421 ) ) ;
#15522=ORIENTED_EDGE ( 'NONE', *, *, #8425, .F. ) ;
#15523=CARTESIAN_POINT ( 'NONE',  ( -25.00000000000000000, -30.00000000000000711, 58.09475019311124555 ) ) ;
#15530=DIRECTION ( 'NONE',  ( 0.000000000000000000, 0.000000000000000000, 1.000000000000000000 ) ) ;
#15534=ORIENTED_EDGE ( 'NONE', *, *, #4751, .F. ) ;
#15536=CARTESIAN_POINT ( 'NONE',  ( 50.00000000000000000, 36.35083268962915781, 50.00000000000000000 ) ) ;
#15541=DIRECTION ( 'NONE',  ( 1.000000000000000000, 0.000000000000000000, 0.000000000000000000 ) ) ;
#15542=CARTESIAN_POINT ( 'NONE',  ( 10.00000000000000178, -164.9999999999999716, 70.00000000000000000 ) ) ;
#15544=LINE ( 'NONE', #10470, #20734 ) ;
#15549=DIRECTION ( 'NONE',  ( 0.000000000000000000, 0.000000000000000000, -1.000000000000000000 ) ) ;
#15552=EDGE_CURVE ( 'NONE', #14202, #18745, #8911, .T. ) ;
#15566=DIRECTION ( 'NONE',  ( 0.000000000000000000, 0.000000000000000000, -1.000000000000000000 ) ) ;
#15571=ADVANCED_FACE ( 'NONE', ( #2869, #4247 ), #11029, .T. ) ;
#15575=ORIENTED_EDGE ( 'NONE', *, *, #19395, .T. ) ;
#15579=VERTEX_POINT ( 'NONE', #6046 ) ;
#15581=CARTESIAN_POINT ( 'NONE',  ( 30.00000000000000000, -50.00000000000000000, -90.00000000000001421 ) ) ;
#15586=DIRECTION ( 'NONE',  ( 0.000000000000000000, -1.000000000000000000, 0.000000000000000000 ) ) ;
#15594=VERTEX_POINT ( 'NONE', #7846 ) ;
#15603=LINE ( 'NONE', #17531, #20175 ) ;
#15606=CARTESIAN_POINT ( 'NONE',  ( -40.00000000000000000, 29.99999999999999289, -120.0000000000000142 ) ) ;
#15609=CIRCLE ( 'NONE', #15958, 3.199999999999994404 ) ;
#15612=ORIENTED_EDGE ( 'NONE', *, *, #15982, .T. ) ;
#15616=EDGE_LOOP ( 'NONE', ( #12207, #5271, #5200, #195 ) ) ;
#15618=LINE ( 'NONE', #1228, #16703 ) ;
#15622=DIRECTION ( 'NONE',  ( -1.000000000000000000, -8.673617379884035472E-17, 0.000000000000000000 ) ) ;
#15629=AXIS2_PLACEMENT_3D ( 'NONE', #6552, #6444, #13234 ) ;
#15633=CARTESIAN_POINT ( 'NONE',  ( 32.34000317368597877, -114.4267062510364354, 75.39615112841575240 ) ) ;
#15644=CARTESIAN_POINT ( 'NONE',  ( 8.948086041649604638, -19.56205492480948038, 76.99190269118484764 ) ) ;
#15653=CARTESIAN_POINT ( 'NONE',  ( 20.06332430260529520, -11.25004336140582417, -82.40911568055234682 ) ) ;
#15658=VECTOR ( 'NONE', #9094, 1000.000000000000000 ) ;
#15663=CARTESIAN_POINT ( 'NONE',  ( 30.00000000000000000, -84.99999999999998579, -75.00000000000001421 ) ) ;
#15672=DIRECTION ( 'NONE',  ( 1.000000000000000000, 0.000000000000000000, 0.000000000000000000 ) ) ;
#15676=ADVANCED_FACE ( 'NONE', ( #14535 ), #7960, .T. ) ;
#15679=AXIS2_PLACEMENT_3D ( 'NONE', #9837, #8058, #16306 ) ;
#15682=CARTESIAN_POINT ( 'NONE',  ( 0.000000000000000000, 0.000000000000000000, -81.99999999999998579 ) ) ;
#15684=CARTESIAN_POINT ( 'NONE',  ( 30.43430782549247837, -42.57363661491096707, -71.38288848018790134 ) ) ;
#15686=ORIENTED_EDGE ( 'NONE', *, *, #6244, .F. ) ;
#15687=EDGE_CURVE ( 'NONE', #4041, #19846, #10952, .T. ) ;
#15698=CARTESIAN_POINT ( 'NONE',  ( -30.00000000000000000, -85.00000000000000000, -11.50000000000000711 ) ) ;
#15701=VECTOR ( 'NONE', #9555, 1000.000000000000000 ) ;
#15703=CIRCLE ( 'NONE', #10289, 2.099999999999997868 ) ;
#15704=VERTEX_POINT ( 'NONE', #11648 ) ;
#15705=CARTESIAN_POINT ( 'NONE',  ( 18.00000000000000000, 0.000000000000000000, -130.0000000000000000 ) ) ;
#15707=EDGE_LOOP ( 'NONE', ( #4007, #17481, #641, #9108, #13439, #8654 ) ) ;
#15709=CARTESIAN_POINT ( 'NONE',  ( 15.62350230547613528, -14.77425901644551764, 73.92464627053533377 ) ) ;
#15715=DIRECTION ( 'NONE',  ( 0.000000000000000000, 0.000000000000000000, -1.000000000000000000 ) ) ;
#15716=EDGE_CURVE ( 'NONE', #19211, #20725, #104, .T. ) ;
#15720=CARTESIAN_POINT ( 'NONE',  ( 48.35276434571220250, -3.649167310370820871, 90.00000000000000000 ) ) ;
#15732=DIRECTION ( 'NONE',  ( 0.000000000000000000, -1.541976423090495387E-16, 1.000000000000000000 ) ) ;
#15733=VERTEX_POINT ( 'NONE', #5073 ) ;
#15736=CARTESIAN_POINT ( 'NONE',  ( -30.00000000000000000, -164.9999999999999716, 50.00000000000001421 ) ) ;
#15738=ORIENTED_EDGE ( 'NONE', *, *, #7035, .F. ) ;
#15741=AXIS2_PLACEMENT_3D ( 'NONE', #13096, #16681, #1962 ) ;
#15743=ORIENTED_EDGE ( 'NONE', *, *, #7411, .F. ) ;
#15745=CARTESIAN_POINT ( 'NONE',  ( 33.70821056661568349, -116.6086985776691876, 76.50504368702979718 ) ) ;
#15752=ORIENTED_EDGE ( 'NONE', *, *, #16961, .F. ) ;
#15758=AXIS2_PLACEMENT_3D ( 'NONE', #4159, #10642, #15923 ) ;
#15761=VERTEX_POINT ( 'NONE', #13042 ) ;
#15762=CARTESIAN_POINT ( 'NONE',  ( 17.42669362192176052, -15.01422997234079126, -79.66264582819448492 ) ) ;
#15764=VECTOR ( 'NONE', #9343, 1000.000000000000000 ) ;
#15765=LINE ( 'NONE', #1266, #17126 ) ;
#15768=ORIENTED_EDGE ( 'NONE', *, *, #433, .F. ) ;
#15770=DIRECTION ( 'NONE',  ( 0.000000000000000000, 0.000000000000000000, -1.000000000000000000 ) ) ;
#15781=ORIENTED_EDGE ( 'NONE', *, *, #9285, .T. ) ;
#15788=AXIS2_PLACEMENT_3D ( 'NONE', #411, #14626, #9755 ) ;
#15793=EDGE_LOOP ( 'NONE', ( #17148, #20181, #6402, #6907 ) ) ;
#15794=CYLINDRICAL_SURFACE ( 'NONE', #9029, 50.00000000000001421 ) ;
#15798=EDGE_CURVE ( 'NONE', #18686, #5413, #4866, .T. ) ;
#15799=AXIS2_PLACEMENT_3D ( 'NONE', #11154, #9358, #15715 ) ;
#15804=CARTESIAN_POINT ( 'NONE',  ( 50.00000000000000000, 4.299168419249259188, 82.52564090190563206 ) ) ;
#15808=AXIS2_PLACEMENT_3D ( 'NONE', #17035, #20421, #14187 ) ;
#15810=VECTOR ( 'NONE', #2425, 1000.000000000000000 ) ;
#15811=DIRECTION ( 'NONE',  ( 0.000000000000000000, 0.000000000000000000, 1.000000000000000000 ) ) ;
#15814=CARTESIAN_POINT ( 'NONE',  ( 19.79075590726360900, -8.422956900484626530, 78.26370100276548669 ) ) ;
#15818=LINE ( 'NONE', #20680, #13226 ) ;
#15820=CARTESIAN_POINT ( 'NONE',  ( 30.00000000000000000, -85.00000000000000000, -1.040949779275250179E-14 ) ) ;
#15822=ORIENTED_EDGE ( 'NONE', *, *, #20027, .F. ) ;
#15823=DIRECTION ( 'NONE',  ( -1.000000000000000000, 0.000000000000000000, 0.000000000000000000 ) ) ;
#15830=CIRCLE ( 'NONE', #15441, 54.99999999999999289 ) ;
#15845=DIRECTION ( 'NONE',  ( 0.000000000000000000, 0.000000000000000000, -1.000000000000000000 ) ) ;
#15850=EDGE_CURVE ( 'NONE', #14887, #18615, #6876, .T. ) ;
#15862=CARTESIAN_POINT ( 'NONE',  ( 10.50529598519903729, -18.76196791309047640, 77.41653794407623934 ) ) ;
#15864=CARTESIAN_POINT ( 'NONE',  ( 30.00000000000000000, -159.9999999999999716, 53.99496054166689873 ) ) ;
#15865=VERTEX_POINT ( 'NONE', #16619 ) ;
#15872=EDGE_LOOP ( 'NONE', ( #16572, #2794 ) ) ;
#15894=DIRECTION ( 'NONE',  ( 1.000000000000000000, 0.000000000000000000, 0.000000000000000000 ) ) ;
#15911=ORIENTED_EDGE ( 'NONE', *, *, #8242, .F. ) ;
#15913=CARTESIAN_POINT ( 'NONE',  ( 20.42938063014384298, -6.725612673823795795, 79.66382435179508548 ) ) ;
#15916=DIRECTION ( 'NONE',  ( 1.000000000000000000, -1.734723475976807094E-16, 0.000000000000000000 ) ) ;
#15920=FACE_OUTER_BOUND ( 'NONE', #5000, .T. ) ;
#15923=DIRECTION ( 'NONE',  ( -1.000000000000000000, 0.000000000000000000, 0.000000000000000000 ) ) ;
#15927=DIRECTION ( 'NONE',  ( 0.000000000000000000, 0.000000000000000000, 1.000000000000000000 ) ) ;
#15928=ORIENTED_EDGE ( 'NONE', *, *, #12075, .T. ) ;
#15931=CIRCLE ( 'NONE', #6784, 2.099999999999990763 ) ;
#15934=DIRECTION ( 'NONE',  ( -1.000000000000000000, -0.000000000000000000, -0.000000000000000000 ) ) ;
#15937=LINE ( 'NONE', #1435, #19511 ) ;
#15942=EDGE_LOOP ( 'NONE', ( #10991, #5375, #968, #7798, #18563, #6610 ) ) ;
#15943=CARTESIAN_POINT ( 'NONE',  ( 10.00000000000000178, -164.9999999999999716, -66.80000000000001137 ) ) ;
#15949=CARTESIAN_POINT ( 'NONE',  ( 50.00000000000000000, 230.0000000000000000, 85.00000000000000000 ) ) ;
#15953=LINE ( 'NONE', #12895, #19065 ) ;
#15958=AXIS2_PLACEMENT_3D ( 'NONE', #12898, #9711, #163 ) ;
#15963=ORIENTED_EDGE ( 'NONE', *, *, #8065, .T. ) ;
#15967=AXIS2_PLACEMENT_3D ( 'NONE', #8914, #12422, #10826 ) ;
#15970=CARTESIAN_POINT ( 'NONE',  ( -30.00000000000000000, -85.00000000000000000, -1.040949779275250179E-14 ) ) ;
#15973=ORIENTED_EDGE ( 'NONE', *, *, #5358, .F. ) ;
#15975=VECTOR ( 'NONE', #16059, 1000.000000000000000 ) ;
#15976=AXIS2_PLACEMENT_3D ( 'NONE', #9345, #4256, #872 ) ;
#15977=DIRECTION ( 'NONE',  ( 0.000000000000000000, -1.000000000000000000, 0.000000000000000000 ) ) ;
#15979=CIRCLE ( 'NONE', #13274, 11.50000000000000000 ) ;
#15982=EDGE_CURVE ( 'NONE', #2747, #5439, #9277, .T. ) ;
#15987=LINE ( 'NONE', #10508, #1724 ) ;
#15988=VECTOR ( 'NONE', #16840, 1000.000000000000000 ) ;
#15990=ORIENTED_EDGE ( 'NONE', *, *, #6397, .T. ) ;
#15991=AXIS2_PLACEMENT_3D ( 'NONE', #4963, #14518, #8045 ) ;
#15993=CARTESIAN_POINT ( 'NONE',  ( 30.00000000000000000, -113.2094389508847314, -74.86138894033632596 ) ) ;
#15997=DIRECTION ( 'NONE',  ( 0.000000000000000000, -1.000000000000000000, 0.000000000000000000 ) ) ;
#15999=CARTESIAN_POINT ( 'NONE',  ( 43.44798870043372574, -10.84402389218931795, -82.73379815179617935 ) ) ;
#16004=CARTESIAN_POINT ( 'NONE',  ( 31.27203855688423673, -112.0327841679104495, -74.37803300064821599 ) ) ;
#16005=EDGE_CURVE ( 'NONE', #10469, #8874, #11298, .T. ) ;
#16011=DIRECTION ( 'NONE',  ( -0.000000000000000000, -0.000000000000000000, 1.000000000000000000 ) ) ;
#16018=FACE_OUTER_BOUND ( 'NONE', #14426, .T. ) ;
#16025=ORIENTED_EDGE ( 'NONE', *, *, #10367, .F. ) ;
#16027=DIRECTION ( 'NONE',  ( -1.734723475976807094E-16, -1.000000000000000000, 0.000000000000000000 ) ) ;
#16032=EDGE_LOOP ( 'NONE', ( #8690, #16930, #10499, #17234 ) ) ;
#16033=CARTESIAN_POINT ( 'NONE',  ( -30.00000000000000000, -97.49621075554985339, -111.6458212409894486 ) ) ;
#16037=DIRECTION ( 'NONE',  ( -1.000000000000000000, -0.000000000000000000, -0.000000000000000000 ) ) ;
#16039=AXIS2_PLACEMENT_3D ( 'NONE', #12841, #1804, #19285 ) ;
#16040=AXIS2_PLACEMENT_3D ( 'NONE', #9269, #4707, #4492 ) ;
#16046=CARTESIAN_POINT ( 'NONE',  ( 40.00000000000000711, -30.00000000000001421, -120.0000000000000142 ) ) ;
#16048=DIRECTION ( 'NONE',  ( 0.000000000000000000, -1.000000000000000000, -8.673617379884036705E-17 ) ) ;
#16051=DIRECTION ( 'NONE',  ( 1.000000000000000000, 0.000000000000000000, 0.000000000000000000 ) ) ;
#16055=ORIENTED_EDGE ( 'NONE', *, *, #6272, .F. ) ;
#16058=EDGE_LOOP ( 'NONE', ( #2351, #6162, #15302, #4846 ) ) ;
#16059=DIRECTION ( 'NONE',  ( -1.000000000000000000, 0.000000000000000000, 0.000000000000000000 ) ) ;
#16063=CARTESIAN_POINT ( 'NONE',  ( -26.35784117651625280, 26.35784117651607872, -130.0000000000000000 ) ) ;
#16072=CARTESIAN_POINT ( 'NONE',  ( 15.54275544017199628, -14.85857375444459905, 79.76610145095158089 ) ) ;
#16073=CIRCLE ( 'NONE', #9648, 20.00000000000000355 ) ;
#16095=EDGE_CURVE ( 'NONE', #14728, #5755, #14409, .T. ) ;
#16096=DIRECTION ( 'NONE',  ( 0.000000000000000000, 0.000000000000000000, 1.000000000000000000 ) ) ;
#16101=EDGE_CURVE ( 'NONE', #12626, #2621, #18078, .T. ) ;
#16107=ORIENTED_EDGE ( 'NONE', *, *, #12098, .F. ) ;
#16111=DIRECTION ( 'NONE',  ( -1.000000000000000000, 0.000000000000000000, 0.000000000000000000 ) ) ;
#16115=CARTESIAN_POINT ( 'NONE',  ( 48.31551312895897610, -3.761933334864634215, -82.40301848942678475 ) ) ;
#16119=CARTESIAN_POINT ( 'NONE',  ( -30.00000000000000000, -124.9999999999999858, 90.00000000000001421 ) ) ;
#16125=DIRECTION ( 'NONE',  ( 0.000000000000000000, 0.000000000000000000, -1.000000000000000000 ) ) ;
#16126=DIRECTION ( 'NONE',  ( -1.000000000000000000, 0.000000000000000000, 0.000000000000000000 ) ) ;
#16133=DIRECTION ( 'NONE',  ( -1.000000000000000000, -0.000000000000000000, -0.000000000000000000 ) ) ;
#16139=CARTESIAN_POINT ( 'NONE',  ( 34.00864524562752678, -27.73747959566527399, 73.62555811687104779 ) ) ;
#16140=AXIS2_PLACEMENT_3D ( 'NONE', #1197, #19604, #11457 ) ;
#16142=ORIENTED_EDGE ( 'NONE', *, *, #5087, .T. ) ;
#16155=CARTESIAN_POINT ( 'NONE',  ( 40.00000000000000711, 39.99999999999998579, -120.0000000000000142 ) ) ;
#16156=ORIENTED_EDGE ( 'NONE', *, *, #18263, .F. ) ;
#16162=ORIENTED_EDGE ( 'NONE', *, *, #17550, .F. ) ;
#16165=CARTESIAN_POINT ( 'NONE',  ( 11.50000000000000000, 1.408343819019456176E-15, -68.00000000000000000 ) ) ;
#16174=DIRECTION ( 'NONE',  ( 0.000000000000000000, 0.000000000000000000, -1.000000000000000000 ) ) ;
#16175=AXIS2_PLACEMENT_3D ( 'NONE', #6921, #13712, #10111 ) ;
#16179=AXIS2_PLACEMENT_3D ( 'NONE', #10142, #8341, #1781 ) ;
#16203=LINE ( 'NONE', #1286, #753 ) ;
#16206=ORIENTED_EDGE ( 'NONE', *, *, #1322, .T. ) ;
#16207=EDGE_CURVE ( 'NONE', #14343, #20337, #13294, .T. ) ;
#16210=CARTESIAN_POINT ( 'NONE',  ( 44.77210880146824223, -9.201386547187325959, -84.14302149088062777 ) ) ;
#16217=CYLINDRICAL_SURFACE ( 'NONE', #15788, 5.000000000000004441 ) ;
#16226=DIRECTION ( 'NONE',  ( 1.000000000000000000, -0.000000000000000000, -0.000000000000000000 ) ) ;
#16235=VERTEX_POINT ( 'NONE', #18204 ) ;
#16240=ORIENTED_EDGE ( 'NONE', *, *, #17268, .F. ) ;
#16243=DIRECTION ( 'NONE',  ( 1.000000000000000000, -0.000000000000000000, -0.000000000000000000 ) ) ;
#16248=DIRECTION ( 'NONE',  ( 1.000000000000000000, 0.000000000000000000, 0.000000000000000000 ) ) ;
#16252=EDGE_LOOP ( 'NONE', ( #20746, #3035, #16385, #19205, #13036, #3433, #13480, #2434, #19903 ) ) ;
#16256=ORIENTED_EDGE ( 'NONE', *, *, #14598, .F. ) ;
#16264=DIRECTION ( 'NONE',  ( 0.000000000000000000, -0.000000000000000000, 1.000000000000000000 ) ) ;
#16279=CARTESIAN_POINT ( 'NONE',  ( 24.99999999999999645, -99.99999999999998579, -52.00000000000000000 ) ) ;
#16288=AXIS2_PLACEMENT_3D ( 'NONE', #4711, #4807, #16051 ) ;
#16291=AXIS2_PLACEMENT_3D ( 'NONE', #10178, #12092, #5302 ) ;
#16303=CIRCLE ( 'NONE', #4459, 2.099999999999990763 ) ;
#16306=DIRECTION ( 'NONE',  ( 1.000000000000000000, 0.000000000000000000, 0.000000000000000000 ) ) ;
#16308=CIRCLE ( 'NONE', #15629, 75.00000000000001421 ) ;
#16310=CARTESIAN_POINT ( 'NONE',  ( 48.36605527348424971, -3.740379660666403261, 82.39768715423042522 ) ) ;
#16311=LINE ( 'NONE', #14934, #16467 ) ;
#16315=VECTOR ( 'NONE', #8992, 1000.000000000000000 ) ;
#16317=AXIS2_PLACEMENT_3D ( 'NONE', #2121, #15054, #321 ) ;
#16331=ORIENTED_EDGE ( 'NONE', *, *, #4033, .T. ) ;
#16337=AXIS2_PLACEMENT_3D ( 'NONE', #5762, #2383, #5665 ) ;
#16341=DIRECTION ( 'NONE',  ( 0.000000000000000000, -0.000000000000000000, 1.000000000000000000 ) ) ;
#16347=CARTESIAN_POINT ( 'NONE',  ( 30.00000000000000000, -39.99999999999999289, 54.09999999999998721 ) ) ;
#16352=DIRECTION ( 'NONE',  ( 0.000000000000000000, 0.000000000000000000, -1.000000000000000000 ) ) ;
#16353=ORIENTED_EDGE ( 'NONE', *, *, #4677, .T. ) ;
#16359=VERTEX_POINT ( 'NONE', #12691 ) ;
#16360=CARTESIAN_POINT ( 'NONE',  ( 50.00000000000000000, 230.0000000000000000, 0.000000000000000000 ) ) ;
#16362=ADVANCED_FACE ( 'NONE', ( #6001 ), #10677, .F. ) ;
#16365=AXIS2_PLACEMENT_3D ( 'NONE', #17, #8081, #3093 ) ;
#16367=DIRECTION ( 'NONE',  ( 1.000000000000000000, 0.000000000000000000, 0.000000000000000000 ) ) ;
#16374=VECTOR ( 'NONE', #8917, 1000.000000000000000 ) ;
#16382=ORIENTED_EDGE ( 'NONE', *, *, #18493, .T. ) ;
#16385=ORIENTED_EDGE ( 'NONE', *, *, #17940, .T. ) ;
#16423=VERTEX_POINT ( 'NONE', #4407 ) ;
#16427=FACE_OUTER_BOUND ( 'NONE', #5633, .T. ) ;
#16439=CIRCLE ( 'NONE', #5596, 11.50000000000000000 ) ;
#16461=VERTEX_POINT ( 'NONE', #8211 ) ;
#16462=DIRECTION ( 'NONE',  ( 0.000000000000000000, 0.000000000000000000, -1.000000000000000000 ) ) ;
#16463=DIRECTION ( 'NONE',  ( 0.000000000000000000, 0.000000000000000000, 1.000000000000000000 ) ) ;
#16465=VERTEX_POINT ( 'NONE', #12802 ) ;
#16467=VECTOR ( 'NONE', #17919, 1000.000000000000000 ) ;
#16469=EDGE_CURVE ( 'NONE', #6600, #14728, #15953, .T. ) ;
#16472=CIRCLE ( 'NONE', #2591, 18.00000000000000000 ) ;
#16484=ORIENTED_EDGE ( 'NONE', *, *, #1614, .F. ) ;
#16485=CIRCLE ( 'NONE', #8700, 54.99999999999999289 ) ;
#16491=CIRCLE ( 'NONE', #18862, 80.00000000000000000 ) ;
#16498=AXIS2_PLACEMENT_3D ( 'NONE', #12182, #12293, #1180 ) ;
#16500=DIRECTION ( 'NONE',  ( 1.000000000000000000, 0.000000000000000000, 0.000000000000000000 ) ) ;
#16524=CARTESIAN_POINT ( 'NONE',  ( 30.00000000000000000, -85.00000000000000000, -1.040949779275250179E-14 ) ) ;
#16527=DIRECTION ( 'NONE',  ( 1.000000000000000000, 0.000000000000000000, 0.000000000000000000 ) ) ;
#16531=DIRECTION ( 'NONE',  ( -1.000000000000000000, 0.000000000000000000, 0.000000000000000000 ) ) ;
#16533=DIRECTION ( 'NONE',  ( 0.000000000000000000, 1.000000000000000000, -8.673617379884034239E-17 ) ) ;
#16535=FACE_OUTER_BOUND ( 'NONE', #3747, .T. ) ;
#16540=CARTESIAN_POINT ( 'NONE',  ( 40.17604362888928904, -15.41257802331652549, 79.36552202533282241 ) ) ;
#16544=SURFACE_STYLE_USAGE ( .BOTH. , #18344 ) ;
#16549=CARTESIAN_POINT ( 'NONE',  ( 34.54863082286252052, -117.7057449628014041, -83.06716769817120394 ) ) ;
#16551=DIRECTION ( 'NONE',  ( 1.000000000000000000, -0.000000000000000000, -0.000000000000000000 ) ) ;
#16552=CARTESIAN_POINT ( 'NONE',  ( -21.35784117651625280, 26.35784117651607872, -120.0000000000000142 ) ) ;
#16553=EDGE_CURVE ( 'NONE', #2556, #9451, #1728, .T. ) ;
#16559=EDGE_LOOP ( 'NONE', ( #7068, #13843, #2273, #6930 ) ) ;
#16560=CARTESIAN_POINT ( 'NONE',  ( 50.00000000000000000, -125.0000000000000000, 90.00000000000002842 ) ) ;
#16572=ORIENTED_EDGE ( 'NONE', *, *, #7027, .T. ) ;
#16573=CARTESIAN_POINT ( 'NONE',  ( 10.00000000000000178, -113.2094389508847314, -74.86138894033631175 ) ) ;
#16580=EDGE_LOOP ( 'NONE', ( #4837, #19913, #15212, #5492 ) ) ;
#16585=EDGE_LOOP ( 'NONE', ( #15990, #6909, #14228, #7354 ) ) ;
#16596=ADVANCED_FACE ( 'NONE', ( #3646 ), #18074, .T. ) ;
#16598=AXIS2_PLACEMENT_3D ( 'NONE', #8916, #10192, #455 ) ;
#16603=EDGE_CURVE ( 'NONE', #16876, #6801, #3540, .T. ) ;
#16611=VERTEX_POINT ( 'NONE', #20060 ) ;
#16615=DIRECTION ( 'NONE',  ( -1.000000000000000000, 0.000000000000000000, 0.000000000000000000 ) ) ;
#16619=CARTESIAN_POINT ( 'NONE',  ( 30.00000000000000000, -40.41646384503856382, 66.42520834682602526 ) ) ;
#16629=LINE ( 'NONE', #14945, #18487 ) ;
#16638=DIRECTION ( 'NONE',  ( -1.000000000000000000, 0.000000000000000000, 0.000000000000000000 ) ) ;
#16639=ORIENTED_EDGE ( 'NONE', *, *, #10266, .F. ) ;
#16641=CARTESIAN_POINT ( 'NONE',  ( 36.99122470214116021, -20.97311120624805625, -70.79638128036988576 ) ) ;
#16642=EDGE_CURVE ( 'NONE', #8495, #6843, #9171, .T. ) ;
#16644=VECTOR ( 'NONE', #14989, 1000.000000000000000 ) ;
#16654=FACE_OUTER_BOUND ( 'NONE', #16032, .T. ) ;
#16658=CARTESIAN_POINT ( 'NONE',  ( -24.99999999999999289, 230.0000000000000000, 84.99999999999998579 ) ) ;
#16661=CARTESIAN_POINT ( 'NONE',  ( -16.87108763463411165, -13.40169213801851278, 74.74090047603390019 ) ) ;
#16668=DIRECTION ( 'NONE',  ( -1.000000000000000000, 0.000000000000000000, 0.000000000000000000 ) ) ;
#16671=VECTOR ( 'NONE', #18286, 1000.000000000000000 ) ;
#16679=AXIS2_PLACEMENT_3D ( 'NONE', #7257, #2297, #4305 ) ;
#16680=EDGE_LOOP ( 'NONE', ( #16882, #17592 ) ) ;
#16681=DIRECTION ( 'NONE',  ( 1.000000000000000000, 0.000000000000000000, 0.000000000000000000 ) ) ;
#16682=CARTESIAN_POINT ( 'NONE',  ( 10.00000000000000178, -40.41646384503850697, -66.42520834682601105 ) ) ;
#16684=CARTESIAN_POINT ( 'NONE',  ( 21.45900938229203447, -1.326995226329880762, -84.99999999999998579 ) ) ;
#16685=ORIENTED_EDGE ( 'NONE', *, *, #12003, .T. ) ;
#16699=CARTESIAN_POINT ( 'NONE',  ( 10.00000000000000178, -113.2094389508847172, 74.86138894033631175 ) ) ;
#16703=VECTOR ( 'NONE', #20498, 1000.000000000000000 ) ;
#16707=VECTOR ( 'NONE', #3103, 1000.000000000000000 ) ;
#16712=VECTOR ( 'NONE', #12979, 1000.000000000000000 ) ;
#16718=ORIENTED_EDGE ( 'NONE', *, *, #3369, .T. ) ;
#16727=ADVANCED_FACE ( 'NONE', ( #18381 ), #3848, .F. ) ;
#16728=AXIS2_PLACEMENT_3D ( 'NONE', #7433, #20475, #11148 ) ;
#16731=DIRECTION ( 'NONE',  ( -1.000000000000000000, 0.000000000000000000, 0.000000000000000000 ) ) ;
#16739=CARTESIAN_POINT ( 'NONE',  ( 30.00000000000000000, -122.0000000000000000, -6.368163355566234804E-15 ) ) ;
#16752=ORIENTED_EDGE ( 'NONE', *, *, #14250, .F. ) ;
#16753=VERTEX_POINT ( 'NONE', #1005 ) ;
#16756=ADVANCED_FACE ( 'NONE', ( #1115 ), #18700, .F. ) ;
#16762=FILL_AREA_STYLE_COLOUR ( '', #11507 ) ;
#16763=CARTESIAN_POINT ( 'NONE',  ( 29.74873734152916782, 24.74873734152916072, -120.0000000000000142 ) ) ;
#16767=AXIS2_PLACEMENT_3D ( 'NONE', #1105, #886, #12010 ) ;
#16768=ORIENTED_EDGE ( 'NONE', *, *, #10045, .T. ) ;
#16772=CARTESIAN_POINT ( 'NONE',  ( -30.00000000000000000, 36.35083268962915781, 50.00000000000000000 ) ) ;
#16778=ORIENTED_EDGE ( 'NONE', *, *, #11038, .F. ) ;
#16785=ORIENTED_EDGE ( 'NONE', *, *, #10912, .T. ) ;
#16786=AXIS2_PLACEMENT_3D ( 'NONE', #15418, #10442, #8833 ) ;
#16787=AXIS2_PLACEMENT_3D ( 'NONE', #19811, #12374, #8679 ) ;
#16793=ORIENTED_EDGE ( 'NONE', *, *, #1991, .F. ) ;
#16797=DIRECTION ( 'NONE',  ( 0.000000000000000000, 0.000000000000000000, 1.000000000000000000 ) ) ;
#16800=ORIENTED_EDGE ( 'NONE', *, *, #15463, .F. ) ;
#16802=VECTOR ( 'NONE', #19904, 1000.000000000000000 ) ;
#16804=DIRECTION ( 'NONE',  ( 1.000000000000000000, 0.000000000000000000, 0.000000000000000000 ) ) ;
#16825=EDGE_LOOP ( 'NONE', ( #20432, #11356 ) ) ;
#16831=ORIENTED_EDGE ( 'NONE', *, *, #8280, .F. ) ;
#16832=DIRECTION ( 'NONE',  ( -1.000000000000000000, 0.000000000000000000, 0.000000000000000000 ) ) ;
#16835=ORIENTED_EDGE ( 'NONE', *, *, #20027, .T. ) ;
#16838=AXIS2_PLACEMENT_3D ( 'NONE', #9068, #13938, #20395 ) ;
#16840=DIRECTION ( 'NONE',  ( -0.000000000000000000, -0.000000000000000000, 1.000000000000000000 ) ) ;
#16845=VECTOR ( 'NONE', #19157, 1000.000000000000000 ) ;
#16865=CARTESIAN_POINT ( 'NONE',  ( -30.00000000000000000, 40.00000000000000000, -120.0000000000000142 ) ) ;
#16871=LINE ( 'NONE', #3619, #8467 ) ;
#16876=VERTEX_POINT ( 'NONE', #7351 ) ;
#16882=ORIENTED_EDGE ( 'NONE', *, *, #6200, .T. ) ;
#16890=DIRECTION ( 'NONE',  ( -0.000000000000000000, 0.000000000000000000, 1.000000000000000000 ) ) ;
#16900=ORIENTED_EDGE ( 'NONE', *, *, #7732, .T. ) ;
#16901=CARTESIAN_POINT ( 'NONE',  ( 21.25854252069020589, -3.402546668908722705, -82.74447975664146782 ) ) ;
#16913=CARTESIAN_POINT ( 'NONE',  ( 50.00000000000000000, 31.35083268962917558, 84.99999999999998579 ) ) ;
#16920=DIRECTION ( 'NONE',  ( 0.000000000000000000, 0.000000000000000000, -1.000000000000000000 ) ) ;
#16930=ORIENTED_EDGE ( 'NONE', *, *, #1322, .F. ) ;
#16940=CIRCLE ( 'NONE', #2054, 200.0000000000000000 ) ;
#16948=FACE_BOUND ( 'NONE', #14411, .T. ) ;
#16957=B_SPLINE_CURVE_WITH_KNOTS ( 'NONE', 3,
 ( #13340, #13542, #10050, #18105, #19987, #13649, #8447, #15029 ),
 .UNSPECIFIED., .F., .F.,
 ( 4, 2, 2, 4 ),
 ( 0.000000000000000000, 0.004499419545982465997, 0.006749129318973705501, 0.008998839091964944137 ),
 .UNSPECIFIED. ) ;
#16958=EDGE_CURVE ( 'NONE', #20075, #16753, #15238, .T. ) ;
#16961=EDGE_CURVE ( 'NONE', #16611, #4158, #6102, .T. ) ;
#16964=VECTOR ( 'NONE', #14183, 1000.000000000000000 ) ;
#16967=LINE ( 'NONE', #4139, #5077 ) ;
#16968=CARTESIAN_POINT ( 'NONE',  ( 24.99999999999999645, -30.00000000000000711, 50.99019513592784847 ) ) ;
#16972=VERTEX_POINT ( 'NONE', #16046 ) ;
#16974=CARTESIAN_POINT ( 'NONE',  ( 10.47959250967882205, -18.77674085041570962, 71.79709706900059984 ) ) ;
#16976=EDGE_LOOP ( 'NONE', ( #8407, #13832, #695, #5373 ) ) ;
#16978=EDGE_LOOP ( 'NONE', ( #15973, #11917, #5392, #9344 ) ) ;
#16979=CARTESIAN_POINT ( 'NONE',  ( 40.00000000000000711, -122.3205080756887639, 80.28096411455982206 ) ) ;
#16987=CIRCLE ( 'NONE', #12253, 21.50000000000000000 ) ;
#16988=DIRECTION ( 'NONE',  ( -0.000000000000000000, -3.469446951953615175E-16, -1.000000000000000000 ) ) ;
#16990=LINE ( 'NONE', #5429, #4883 ) ;
#16995=ORIENTED_EDGE ( 'NONE', *, *, #12003, .F. ) ;
#16999=AXIS2_PLACEMENT_3D ( 'NONE', #4334, #18753, #10800 ) ;
#17000=CARTESIAN_POINT ( 'NONE',  ( -9.587454675490699074, -19.24766271911510529, -71.57389447320451836 ) ) ;
#17002=VERTEX_POINT ( 'NONE', #16347 ) ;
#17009=ORIENTED_EDGE ( 'NONE', *, *, #3395, .F. ) ;
#17010=DIRECTION ( 'NONE',  ( 1.000000000000000000, 0.000000000000000000, 0.000000000000000000 ) ) ;
#17013=ORIENTED_EDGE ( 'NONE', *, *, #18666, .F. ) ;
#17015=EDGE_CURVE ( 'NONE', #15594, #5687, #9630, .T. ) ;
#17017=CIRCLE ( 'NONE', #6846, 80.00000000000000000 ) ;
#17022=AXIS2_PLACEMENT_3D ( 'NONE', #13627, #2290, #13734 ) ;
#17028=CARTESIAN_POINT ( 'NONE',  ( -11.45434770231475596, -18.20738947644333550, 77.71966828574345243 ) ) ;
#17029=AXIS2_PLACEMENT_3D ( 'NONE', #4025, #12193, #10405 ) ;
#17031=FACE_OUTER_BOUND ( 'NONE', #18724, .T. ) ;
#17032=CIRCLE ( 'NONE', #19406, 3.199999999999994404 ) ;
#17034=ORIENTED_EDGE ( 'NONE', *, *, #13240, .F. ) ;
#17035=CARTESIAN_POINT ( 'NONE',  ( -24.99999999999999645, -97.49621075554985339, -111.6458212409894486 ) ) ;
#17038=CARTESIAN_POINT ( 'NONE',  ( -7.494266837154794914, -21.79755816881963781, -75.89910374996922826 ) ) ;
#17042=ORIENTED_EDGE ( 'NONE', *, *, #13253, .T. ) ;
#17045=DIRECTION ( 'NONE',  ( -1.000000000000000000, 0.000000000000000000, 0.000000000000000000 ) ) ;
#17056=EDGE_CURVE ( 'NONE', #9376, #14238, #16871, .T. ) ;
#17065=CARTESIAN_POINT ( 'NONE',  ( 30.00000000000000000, -49.99999999999999289, -71.93747284969079203 ) ) ;
#17072=CARTESIAN_POINT ( 'NONE',  ( 34.33484195354434831, -26.68654532909942745, -68.63850682271649362 ) ) ;
#17074=VERTEX_POINT ( 'NONE', #5316 ) ;
#17076=AXIS2_PLACEMENT_3D ( 'NONE', #20594, #3004, #14356 ) ;
#17080=VECTOR ( 'NONE', #10491, 1000.000000000000000 ) ;
#17082=EDGE_CURVE ( 'NONE', #10203, #16753, #15175, .T. ) ;
#17089=EDGE_LOOP ( 'NONE', ( #1523, #6299, #4369, #6847 ) ) ;
#17091=CARTESIAN_POINT ( 'NONE',  ( -21.45900938229203447, -1.326995226329893862, 84.99999999999998579 ) ) ;
#17092=ORIENTED_EDGE ( 'NONE', *, *, #17213, .F. ) ;
#17093=ADVANCED_FACE ( 'NONE', ( #16654 ), #2141, .F. ) ;
#17096=LINE ( 'NONE', #2579, #360 ) ;
#17098=DIRECTION ( 'NONE',  ( 1.000000000000000000, 0.000000000000000000, 0.000000000000000000 ) ) ;
#17099=ORIENTED_EDGE ( 'NONE', *, *, #5172, .F. ) ;
#17102=DIRECTION ( 'NONE',  ( 0.000000000000000000, 0.000000000000000000, -1.000000000000000000 ) ) ;
#17104=DIRECTION ( 'NONE',  ( -0.000000000000000000, -3.469446951953614682E-16, -1.000000000000000000 ) ) ;
#17105=EDGE_CURVE ( 'NONE', #18656, #12982, #557, .T. ) ;
#17112=CARTESIAN_POINT ( 'NONE',  ( 13.23800900960920401, -16.95692081615698044, -72.71034110640576387 ) ) ;
#17113=LINE ( 'NONE', #17324, #4161 ) ;
#17115=ORIENTED_EDGE ( 'NONE', *, *, #4027, .T. ) ;
#17119=ORIENTED_EDGE ( 'NONE', *, *, #19834, .F. ) ;
#17123=FACE_OUTER_BOUND ( 'NONE', #3202, .T. ) ;
#17126=VECTOR ( 'NONE', #1366, 1000.000000000000000 ) ;
#17131=CIRCLE ( 'NONE', #19827, 21.50000000000000000 ) ;
#17139=EDGE_CURVE ( 'NONE', #2408, #1189, #7642, .T. ) ;
#17143=VECTOR ( 'NONE', #16531, 1000.000000000000000 ) ;
#17147=DIRECTION ( 'NONE',  ( -0.000000000000000000, -1.000000000000000000, -0.000000000000000000 ) ) ;
#17148=ORIENTED_EDGE ( 'NONE', *, *, #8280, .T. ) ;
#17149=CARTESIAN_POINT ( 'NONE',  ( 10.34366295437100014, -20.54632100680313656, -76.49602251636484596 ) ) ;
#17154=ORIENTED_EDGE ( 'NONE', *, *, #166, .F. ) ;
#17156=VERTEX_POINT ( 'NONE', #15698 ) ;
#17157=DIRECTION ( 'NONE',  ( 1.000000000000000000, -0.000000000000000000, -0.000000000000000000 ) ) ;
#17173=VERTEX_POINT ( 'NONE', #18667 ) ;
#17179=CYLINDRICAL_SURFACE ( 'NONE', #14632, 2.099999999999997868 ) ;
#17184=B_SPLINE_CURVE_WITH_KNOTS ( 'NONE', 3,
 ( #2092, #18524, #19986, #3987, #2196, #5469, #18211, #2404, #12155, #7273, #5371, #13541, #7061, #8863, #3771, #3675, #18622, #5269, #1997, #11839, #10049, #8548, #18306, #10254 ),
 .UNSPECIFIED., .F., .F.,
 ( 4, 2, 2, 2, 2, 2, 2, 2, 2, 2, 2, 4 ),
 ( 1.430489624538199204E-17, 0.002868008191885854877, 0.005736016383771695010, 0.007170020479714604884, 0.008604024575657518228, 0.01147203276754338135, 0.01290603686348630076, 0.01434004095942921671, 0.01720804915131499135, 0.02007605734320076774, 0.02151006143914363511, 0.02294406553508650942 ),
 .UNSPECIFIED. ) ;
#17190=AXIS2_PLACEMENT_3D ( 'NONE', #15542, #17147, #14079 ) ;
#17194=DIRECTION ( 'NONE',  ( -0.000000000000000000, -0.000000000000000000, 1.000000000000000000 ) ) ;
#17199=DIRECTION ( 'NONE',  ( 0.000000000000000000, -8.673617379884034239E-17, -1.000000000000000000 ) ) ;
#17204=DIRECTION ( 'NONE',  ( -1.000000000000000000, 0.000000000000000000, 0.000000000000000000 ) ) ;
#17205=ORIENTED_EDGE ( 'NONE', *, *, #8071, .T. ) ;
#17210=CARTESIAN_POINT ( 'NONE',  ( 11.50000000000000000, 0.000000000000000000, 68.00000000000000000 ) ) ;
#17213=EDGE_CURVE ( 'NONE', #20537, #18745, #9235, .T. ) ;
#17216=DIRECTION ( 'NONE',  ( -0.000000000000000000, -0.000000000000000000, 1.000000000000000000 ) ) ;
#17224=PLANE ( 'NONE',  #4868 ) ;
#17234=ORIENTED_EDGE ( 'NONE', *, *, #12609, .T. ) ;
#17240=ORIENTED_EDGE ( 'NONE', *, *, #3710, .T. ) ;
#17241=ADVANCED_FACE ( 'NONE', ( #2449 ), #7530, .F. ) ;
#17244=CARTESIAN_POINT ( 'NONE',  ( -10.86880604054440269, -18.56337176816380108, 77.52347650517093314 ) ) ;
#17248=EDGE_CURVE ( 'NONE', #1656, #11513, #8070, .T. ) ;
#17254=CARTESIAN_POINT ( 'NONE',  ( -21.45900938229203447, -1.326995226329893862, 84.99999999999998579 ) ) ;
#17255=CARTESIAN_POINT ( 'NONE',  ( 56.98610214956098474, -164.9999999999999716, -84.54208835637706443 ) ) ;
#17260=CYLINDRICAL_SURFACE ( 'NONE', #12604, 2.099999999999997868 ) ;
#17265=EDGE_CURVE ( 'NONE', #5277, #6801, #8494, .T. ) ;
#17266=AXIS2_PLACEMENT_3D ( 'NONE', #2488, #8948, #15413 ) ;
#17267=PRODUCT_DEFINITION_CONTEXT ( 'detailed design', #18609, 'design' ) ;
#17268=EDGE_CURVE ( 'NONE', #4973, #17868, #17610, .T. ) ;
#17273=ADVANCED_FACE ( 'NONE', ( #14539 ), #20885, .F. ) ;
#17279=VERTEX_POINT ( 'NONE', #14223 ) ;
#17284=DIRECTION ( 'NONE',  ( 1.000000000000000000, -0.000000000000000000, -0.000000000000000000 ) ) ;
#17287=CARTESIAN_POINT ( 'NONE',  ( 39.24980374687644513, -121.8707082894959939, -79.92871449913415915 ) ) ;
#17289=AXIS2_PLACEMENT_3D ( 'NONE', #20138, #1380, #19270 ) ;
#17291=EDGE_CURVE ( 'NONE', #18936, #5467, #51, .T. ) ;
#17306=DIRECTION ( 'NONE',  ( -1.000000000000000000, 0.000000000000000000, 0.000000000000000000 ) ) ;
#17309=PLANE ( 'NONE',  #19546 ) ;
#17311=ORIENTED_EDGE ( 'NONE', *, *, #6796, .F. ) ;
#17312=CARTESIAN_POINT ( 'NONE',  ( -39.99999999999999289, -30.00000000000000000, -120.0000000000000142 ) ) ;
#17313=LINE ( 'NONE', #17428, #11061 ) ;
#17317=AXIS2_PLACEMENT_3D ( 'NONE', #4123, #2230, #8900 ) ;
#17318=ORIENTED_EDGE ( 'NONE', *, *, #2110, .F. ) ;
#17323=DIRECTION ( 'NONE',  ( 0.000000000000000000, 0.000000000000000000, -1.000000000000000000 ) ) ;
#17324=CARTESIAN_POINT ( 'NONE',  ( 30.00000000000000000, -110.0000000000000142, -1.426443885047873890E-14 ) ) ;
#17331=AXIS2_PLACEMENT_3D ( 'NONE', #18635, #4100, #5586 ) ;
#17338=EDGE_LOOP ( 'NONE', ( #3449, #6720, #17042, #4397 ) ) ;
#17340=CARTESIAN_POINT ( 'NONE',  ( -25.00000000000000000, -30.00000000000000711, 58.09475019311124555 ) ) ;
#17354=CARTESIAN_POINT ( 'NONE',  ( 30.00000000000000000, -30.00000000000000711, 58.09475019311124555 ) ) ;
#17359=CYLINDRICAL_SURFACE ( 'NONE', #3133, 80.00000000000000000 ) ;
#17361=LINE ( 'NONE', #9414, #20352 ) ;
#17367=DIRECTION ( 'NONE',  ( 0.000000000000000000, 0.000000000000000000, -1.000000000000000000 ) ) ;
#17375=VERTEX_POINT ( 'NONE', #14333 ) ;
#17377=PLANE ( 'NONE',  #11098 ) ;
#17381=B_SPLINE_CURVE_WITH_KNOTS ( 'NONE', 3,
 ( #6342, #982, #12827, #7425 ),
 .UNSPECIFIED., .F., .F.,
 ( 4, 4 ),
 ( 6.938893903907228378E-18, 0.005429897942433492726 ),
 .UNSPECIFIED. ) ;
#17385=CIRCLE ( 'NONE', #20069, 5.000000000000004441 ) ;
#17386=ORIENTED_EDGE ( 'NONE', *, *, #5731, .T. ) ;
#17389=ORIENTED_EDGE ( 'NONE', *, *, #6746, .T. ) ;
#17390=CARTESIAN_POINT ( 'NONE',  ( 41.73623995412758347, -13.12544047974070693, -80.94893887662107090 ) ) ;
#17395=LINE ( 'NONE', #15581, #15459 ) ;
#17400=DIRECTION ( 'NONE',  ( 1.000000000000000000, 0.000000000000000000, 0.000000000000000000 ) ) ;
#17410=LINE ( 'NONE', #2877, #15764 ) ;
#17411=ADVANCED_FACE ( 'NONE', ( #7723, #14196, #4536, #4099, #837, #5916 ), #14087, .T. ) ;
#17417=CARTESIAN_POINT ( 'NONE',  ( 20.23544477270224817, -7.290198706429656283, 79.18558687180568256 ) ) ;
#17418=ORIENTED_EDGE ( 'NONE', *, *, #13711, .T. ) ;
#17423=DIRECTION ( 'NONE',  ( 0.000000000000000000, 0.000000000000000000, -1.000000000000000000 ) ) ;
#17427=DIRECTION ( 'NONE',  ( -0.000000000000000000, -0.000000000000000000, 1.000000000000000000 ) ) ;
#17428=CARTESIAN_POINT ( 'NONE',  ( 50.00000000000000000, 31.35083268962912584, 6.892027480330899929E-14 ) ) ;
#17433=ORIENTED_EDGE ( 'NONE', *, *, #6105, .T. ) ;
#17438=CARTESIAN_POINT ( 'NONE',  ( 50.00000000000000000, -159.9999999999999716, 85.00000000000000000 ) ) ;
#17442=CARTESIAN_POINT ( 'NONE',  ( 24.99999999999999645, -122.0000000000000000, -6.368163355566234804E-15 ) ) ;
#17446=LINE ( 'NONE', #15523, #3462 ) ;
#17450=CARTESIAN_POINT ( 'NONE',  ( -11.50000000000000000, 0.000000000000000000, -68.00000000000000000 ) ) ;
#17459=ORIENTED_EDGE ( 'NONE', *, *, #8425, .T. ) ;
#17460=CARTESIAN_POINT ( 'NONE',  ( 16.19442412633312856, -14.14534473583932339, 80.24994515060548395 ) ) ;
#17465=FACE_OUTER_BOUND ( 'NONE', #2546, .T. ) ;
#17469=AXIS2_PLACEMENT_3D ( 'NONE', #1404, #10932, #12201 ) ;
#17481=ORIENTED_EDGE ( 'NONE', *, *, #11308, .T. ) ;
#17489=CARTESIAN_POINT ( 'NONE',  ( -30.00000000000000000, 40.00000000000000000, -130.0000000000000000 ) ) ;
#17490=VECTOR ( 'NONE', #544, 1000.000000000000000 ) ;
#17493=ORIENTED_EDGE ( 'NONE', *, *, #11447, .F. ) ;
#17497=CARTESIAN_POINT ( 'NONE',  ( 31.56332346631016961, -35.94799839343871639, -71.81695530636427804 ) ) ;
#17499=AXIS2_PLACEMENT_3D ( 'NONE', #719, #13764, #17045 ) ;
#17523=CARTESIAN_POINT ( 'NONE',  ( 21.25854252069020234, -3.402546668908731586, 82.74447975664143939 ) ) ;
#17524=ADVANCED_FACE ( 'NONE', ( #10798 ), #17260, .F. ) ;
#17527=LINE ( 'NONE', #2996, #17743 ) ;
#17531=CARTESIAN_POINT ( 'NONE',  ( -30.00000000000000000, -40.00000000000000000, -120.0000000000000142 ) ) ;
#17544=EDGE_CURVE ( 'NONE', #11718, #10704, #9625, .T. ) ;
#17548=LINE ( 'NONE', #14364, #4398 ) ;
#17550=EDGE_CURVE ( 'NONE', #4504, #14189, #19031, .T. ) ;
#17559=CARTESIAN_POINT ( 'NONE',  ( 50.00000000000000000, -151.4095880458873467, -44.60680010464253087 ) ) ;
#17562=EDGE_CURVE ( 'NONE', #5841, #20820, #9513, .T. ) ;
#17568=ORIENTED_EDGE ( 'NONE', *, *, #15265, .T. ) ;
#17569=DIRECTION ( 'NONE',  ( 0.000000000000000000, 0.000000000000000000, -1.000000000000000000 ) ) ;
#17576=CARTESIAN_POINT ( 'NONE',  ( 10.00000000000000178, -164.9999999999999716, -73.20000000000000284 ) ) ;
#17592=ORIENTED_EDGE ( 'NONE', *, *, #7421, .T. ) ;
#17597=ORIENTED_EDGE ( 'NONE', *, *, #9374, .F. ) ;
#17610=LINE ( 'NONE', #15804, #2422 ) ;
#17631=CARTESIAN_POINT ( 'NONE',  ( -44.00000000000000000, -85.00000000000000000, -11.50000000000000711 ) ) ;
#17635=CARTESIAN_POINT ( 'NONE',  ( 50.00000000000000000, -159.9999999999999716, -85.00000000000000000 ) ) ;
#17637=CARTESIAN_POINT ( 'NONE',  ( -24.99999999999999289, -85.00000000000000000, -1.040949779275250179E-14 ) ) ;
#17640=LINE ( 'NONE', #1333, #5884 ) ;
#17641=DIRECTION ( 'NONE',  ( 0.000000000000000000, 0.000000000000000000, -1.000000000000000000 ) ) ;
#17643=CARTESIAN_POINT ( 'NONE',  ( 30.00000000000000000, -122.0000000000000000, -6.368163355566234804E-15 ) ) ;
#17647=EDGE_CURVE ( 'NONE', #5928, #17279, #1096, .T. ) ;
#17648=CARTESIAN_POINT ( 'NONE',  ( 11.50000000000000000, 1.408343819019456176E-15, -81.99999999999998579 ) ) ;
#17655=CARTESIAN_POINT ( 'NONE',  ( 30.00000000000000000, -85.00000000000000000, -1.040949779275250179E-14 ) ) ;
#17656=ADVANCED_FACE ( 'NONE', ( #8647 ), #10352, .T. ) ;
#17658=AXIS2_PLACEMENT_3D ( 'NONE', #11140, #19289, #6 ) ;
#17664=VECTOR ( 'NONE', #6766, 1000.000000000000000 ) ;
#17669=LINE ( 'NONE', #15864, #209 ) ;
#17674=CARTESIAN_POINT ( 'NONE',  ( 24.99999999999999645, -122.0000000000000000, -2.100000000000004086 ) ) ;
#17677=DIRECTION ( 'NONE',  ( 1.000000000000000000, 0.000000000000000000, 0.000000000000000000 ) ) ;
#17682=FACE_BOUND ( 'NONE', #2594, .T. ) ;
#17684=CARTESIAN_POINT ( 'NONE',  ( 50.00000000000000000, 36.35083268962920044, -90.00000000000000000 ) ) ;
#17689=CARTESIAN_POINT ( 'NONE',  ( 30.00000000000000000, -39.99999999999999289, -52.00000000000000000 ) ) ;
#17696=CLOSED_SHELL ( 'NONE', ( #15437, #3, #2901, #18280, #11181, #17524, #3024, #12876, #11077, #818, #19091, #1038, #1978, #3506, #86, #7450, #5447, #19292, #15676, #3520, #8913, #55, #6047, #11911, #12712, #12364, #3429, #6906, #17411, #4845, #7788, #16727, #16596, #10006, #7935, #11806, #3597, #14185, #4566, #12519, #18961, #15076, #895, #4904, #3233, #8304, #19865, #13750, #9753, #1599, #18919, #20470, #2708, #5929, #11687, #19357, #9577, #5317, #17656, #15571, #12670, #10504, #10088, #15506, #4574, #12621, #17802, #3380, #14682, #4301, #5, #20495, #15471, #6691, #20463, #5045, #16362, #20809, #18407, #17241, #19451, #534, #20063, #5254, #8169, #8816, #20927, #3262, #12739, #19596, #2504, #10295, #12986, #6311, #8971, #9918, #236, #5570, #11710, #19456, #2066, #8445, #10453, #13336, #2479, #13529, #10148, #436, #3270, #11779, #14219, #7825, #18642, #9628, #20329, #922, #6511, #13978, #17273, #11055, #732, #18032, #14628, #17093, #12865, #7243, #2627, #13190, #16756 ) ) ;
#17700=CIRCLE ( 'NONE', #7527, 2.099999999999997868 ) ;
#17702=FACE_OUTER_BOUND ( 'NONE', #12018, .T. ) ;
#17704=CARTESIAN_POINT ( 'NONE',  ( 10.00000000000000178, -164.9999999999999716, -70.00000000000000000 ) ) ;
#17705=CARTESIAN_POINT ( 'NONE',  ( -24.99999999999999289, -30.00000000000000711, -50.99019513592786268 ) ) ;
#17707=AXIS2_PLACEMENT_3D ( 'NONE', #1353, #1027, #18725 ) ;
#17719=CARTESIAN_POINT ( 'NONE',  ( 30.00000000000000000, -85.00000000000000000, 74.99999999999998579 ) ) ;
#17726=LINE ( 'NONE', #1522, #14043 ) ;
#17732=CARTESIAN_POINT ( 'NONE',  ( 50.00000000000000000, 230.0000000000000000, 0.000000000000000000 ) ) ;
#17733=CARTESIAN_POINT ( 'NONE',  ( 30.00000000000000000, -50.00000000000000000, 71.93747284969079203 ) ) ;
#17735=ORIENTED_EDGE ( 'NONE', *, *, #19234, .F. ) ;
#17742=AXIS2_PLACEMENT_3D ( 'NONE', #9466, #12663, #14244 ) ;
#17743=VECTOR ( 'NONE', #20478, 1000.000000000000000 ) ;
#17745=VECTOR ( 'NONE', #4607, 1000.000000000000000 ) ;
#17750=EDGE_CURVE ( 'NONE', #10368, #12982, #19020, .T. ) ;
#17751=VERTEX_POINT ( 'NONE', #18939 ) ;
#17756=ORIENTED_EDGE ( 'NONE', *, *, #18042, .T. ) ;
#17763=VECTOR ( 'NONE', #1716, 1000.000000000000000 ) ;
#17765=DIRECTION ( 'NONE',  ( 0.000000000000000000, 1.000000000000000000, 0.000000000000000000 ) ) ;
#17768=DIRECTION ( 'NONE',  ( 1.000000000000000000, -0.000000000000000000, 0.000000000000000000 ) ) ;
#17772=EDGE_CURVE ( 'NONE', #11773, #4597, #1703, .T. ) ;
#17776=CYLINDRICAL_SURFACE ( 'NONE', #14485, 21.50000000000000000 ) ;
#17778=ORIENTED_EDGE ( 'NONE', *, *, #12180, .T. ) ;
#17795=CARTESIAN_POINT ( 'NONE',  ( 30.00000000000000000, -85.00000000000000000, -1.040949779275250179E-14 ) ) ;
#17800=DIRECTION ( 'NONE',  ( -1.000000000000000000, 0.000000000000000000, 0.000000000000000000 ) ) ;
#17802=ADVANCED_FACE ( 'NONE', ( #13100 ), #18182, .F. ) ;
#17809=ORIENTED_EDGE ( 'NONE', *, *, #20751, .T. ) ;
#17821=CIRCLE ( 'NONE', #18472, 11.50000000000000000 ) ;
#17827=LINE ( 'NONE', #17719, #13179 ) ;
#17833=DIRECTION ( 'NONE',  ( -0.000000000000000000, 0.000000000000000000, -1.000000000000000000 ) ) ;
#17835=CARTESIAN_POINT ( 'NONE',  ( -24.99999999999999289, -127.3290820621008379, -85.00000000000000000 ) ) ;
#17843=ORIENTED_EDGE ( 'NONE', *, *, #5155, .F. ) ;
#17846=DIRECTION ( 'NONE',  ( 0.000000000000000000, 0.000000000000000000, -1.000000000000000000 ) ) ;
#17850=VERTEX_POINT ( 'NONE', #3542 ) ;
#17858=DIRECTION ( 'NONE',  ( 1.000000000000000000, 0.000000000000000000, 0.000000000000000000 ) ) ;
#17861=CIRCLE ( 'NONE', #3957, 5.000000000000004441 ) ;
#17865=DIRECTION ( 'NONE',  ( 1.000000000000000000, -0.000000000000000000, -0.000000000000000000 ) ) ;
#17866=EDGE_CURVE ( 'NONE', #19846, #9320, #6931, .T. ) ;
#17868=VERTEX_POINT ( 'NONE', #5034 ) ;
#17871=CARTESIAN_POINT ( 'NONE',  ( -44.00000000000000000, -85.00000000000000000, -1.040949779275250179E-14 ) ) ;
#17875=ORIENTED_EDGE ( 'NONE', *, *, #4093, .F. ) ;
#17877=ORIENTED_EDGE ( 'NONE', *, *, #16005, .F. ) ;
#17887=CARTESIAN_POINT ( 'NONE',  ( -19.21120049922023298, -12.66361362969373872, -81.30997835302029841 ) ) ;
#17891=CARTESIAN_POINT ( 'NONE',  ( -24.99999999999999289, -170.8299878242309546, -15.48896927112552824 ) ) ;
#17894=CARTESIAN_POINT ( 'NONE',  ( -44.00000000000000000, -85.00000000000000000, -14.50000000000000533 ) ) ;
#17904=VERTEX_POINT ( 'NONE', #59 ) ;
#17907=CARTESIAN_POINT ( 'NONE',  ( 45.22159793441012710, -8.673994507468377080, 78.07221698934969822 ) ) ;
#17908=VERTEX_POINT ( 'NONE', #8416 ) ;
#17911=ORIENTED_EDGE ( 'NONE', *, *, #8798, .F. ) ;
#17912=DIRECTION ( 'NONE',  ( 0.000000000000000000, 0.000000000000000000, -1.000000000000000000 ) ) ;
#17914=ORIENTED_EDGE ( 'NONE', *, *, #19914, .T. ) ;
#17919=DIRECTION ( 'NONE',  ( 0.000000000000000000, 0.000000000000000000, 1.000000000000000000 ) ) ;
#17922=EDGE_CURVE ( 'NONE', #20752, #1213, #8386, .T. ) ;
#17936=CARTESIAN_POINT ( 'NONE',  ( 30.11828614405466809, -45.99142187292924433, 71.48965128677856740 ) ) ;
#17940=EDGE_CURVE ( 'NONE', #15306, #8783, #5398, .T. ) ;
#17943=ORIENTED_EDGE ( 'NONE', *, *, #820, .T. ) ;
#17946=LINE ( 'NONE', #11270, #149 ) ;
#17947=LINE ( 'NONE', #16155, #1155 ) ;
#17950=ORIENTED_EDGE ( 'NONE', *, *, #19395, .F. ) ;
#17958=ORIENTED_EDGE ( 'NONE', *, *, #16101, .T. ) ;
#17961=CARTESIAN_POINT ( 'NONE',  ( -24.99999999999999289, -113.2094389508847314, -74.86138894033631175 ) ) ;
#17965=ORIENTED_EDGE ( 'NONE', *, *, #6858, .F. ) ;
#17969=ORIENTED_EDGE ( 'NONE', *, *, #10367, .T. ) ;
#17970=CARTESIAN_POINT ( 'NONE',  ( -21.45900938229203447, -1.326995226329880762, -84.99999999999998579 ) ) ;
#17980=PLANE ( 'NONE',  #13059 ) ;
#17982=EDGE_CURVE ( 'NONE', #18338, #20337, #17548, .T. ) ;
#17984=DIRECTION ( 'NONE',  ( -0.000000000000000000, 0.7812527682501551052, 0.6242147964454779485 ) ) ;
#17986=AXIS2_PLACEMENT_3D ( 'NONE', #7885, #14367, #1739 ) ;
#17995=DIRECTION ( 'NONE',  ( -0.000000000000000000, -0.000000000000000000, 1.000000000000000000 ) ) ;
#17996=DIRECTION ( 'NONE',  ( 1.000000000000000000, 0.000000000000000000, 0.000000000000000000 ) ) ;
#17997=CARTESIAN_POINT ( 'NONE',  ( 31.90258477071211729, -34.42335243099921627, 66.95649890984037711 ) ) ;
#17998=EDGE_LOOP ( 'NONE', ( #19232, #12009, #7069, #14323, #12671, #7349, #11374, #7688, #13725, #4395, #9425, #7986, #7994, #16768, #8423, #18241, #15230, #7990, #12723, #15481 ) ) ;
#17999=VECTOR ( 'NONE', #13624, 1000.000000000000000 ) ;
#18006=CIRCLE ( 'NONE', #5134, 3.199999999999994404 ) ;
#18009=EDGE_CURVE ( 'NONE', #1571, #6843, #9377, .T. ) ;
#18019=DIRECTION ( 'NONE',  ( 0.000000000000000000, 0.000000000000000000, -1.000000000000000000 ) ) ;
#18023=EDGE_CURVE ( 'NONE', #5556, #8714, #7566, .T. ) ;
#18027=ORIENTED_EDGE ( 'NONE', *, *, #19581, .F. ) ;
#18032=ADVANCED_FACE ( 'NONE', ( #10762 ), #17224, .T. ) ;
#18041=CARTESIAN_POINT ( 'NONE',  ( 40.00000000000000000, -122.3205080756887639, 86.97287527660684248 ) ) ;
#18042=EDGE_CURVE ( 'NONE', #3964, #1999, #12553, .T. ) ;
#18056=CARTESIAN_POINT ( 'NONE',  ( 8.500000000000000000, 1.040949779275250140E-15, -90.00000000000000000 ) ) ;
#18059=DIRECTION ( 'NONE',  ( -1.000000000000000000, -0.000000000000000000, -0.000000000000000000 ) ) ;
#18061=CARTESIAN_POINT ( 'NONE',  ( -30.00000000000000000, -85.00000000000000000, -1.040949779275250179E-14 ) ) ;
#18063=EDGE_CURVE ( 'NONE', #14211, #9434, #15618, .T. ) ;
#18064=CIRCLE ( 'NONE', #4518, 80.00000000000000000 ) ;
#18065=EDGE_LOOP ( 'NONE', ( #12378, #1351, #744, #7198 ) ) ;
#18070=CARTESIAN_POINT ( 'NONE',  ( 50.00000000000000000, -3.649167310370807105, -90.00000000000000000 ) ) ;
#18072=ORIENTED_EDGE ( 'NONE', *, *, #4302, .F. ) ;
#18074=CYLINDRICAL_SURFACE ( 'NONE', #3730, 55.00000000000000711 ) ;
#18078=CIRCLE ( 'NONE', #20778, 2.099999999999990763 ) ;
#18088=CARTESIAN_POINT ( 'NONE',  ( 30.00000000000000000, -151.4095880458873467, -44.60680010464253087 ) ) ;
#18089=EDGE_CURVE ( 'NONE', #20282, #19655, #9605, .T. ) ;
#18093=CARTESIAN_POINT ( 'NONE',  ( 50.00000000000000000, 4.299168419249266293, -84.99999999999998579 ) ) ;
#18096=ORIENTED_EDGE ( 'NONE', *, *, #274, .T. ) ;
#18104=FACE_OUTER_BOUND ( 'NONE', #20473, .T. ) ;
#18105=CARTESIAN_POINT ( 'NONE',  ( 42.80822997663166518, -124.2670557317275382, -81.91943786100384273 ) ) ;
#18109=VECTOR ( 'NONE', #15466, 1000.000000000000000 ) ;
#18110=FACE_BOUND ( 'NONE', #10401, .T. ) ;
#18114=ORIENTED_EDGE ( 'NONE', *, *, #17750, .F. ) ;
#18132=EDGE_LOOP ( 'NONE', ( #19241, #2289, #2152, #9790 ) ) ;
#18133=CARTESIAN_POINT ( 'NONE',  ( 50.00000000000000000, -127.3290820621008947, -85.00000000000000000 ) ) ;
#18136=CARTESIAN_POINT ( 'NONE',  ( 30.00000000000000000, -113.2094389508847314, 74.86138894033629754 ) ) ;
#18137=AXIS2_PLACEMENT_3D ( 'NONE', #15970, #4947, #5042 ) ;
#18142=EDGE_CURVE ( 'NONE', #17904, #16972, #17640, .T. ) ;
#18147=CARTESIAN_POINT ( 'NONE',  ( 35.67727064648033064, -118.9655047900900371, -84.00146531284171658 ) ) ;
#18150=LINE ( 'NONE', #16763, #4766 ) ;
#18160=FACE_OUTER_BOUND ( 'NONE', #20094, .T. ) ;
#18164=CIRCLE ( 'NONE', #15118, 21.50000000000000000 ) ;
#18165=ORIENTED_EDGE ( 'NONE', *, *, #4017, .T. ) ;
#18167=CIRCLE ( 'NONE', #18857, 2.099999999999997868 ) ;
#18170=EDGE_CURVE ( 'NONE', #10552, #11331, #1648, .T. ) ;
#18171=AXIS2_PLACEMENT_3D ( 'NONE', #13138, #20861, #19585 ) ;
#18172=MECHANICAL_DESIGN_GEOMETRIC_PRESENTATION_REPRESENTATION('',(#10737),#4632);
#18174=CARTESIAN_POINT ( 'NONE',  ( -30.00000000000000000, -85.00000000000000000, -1.040949779275250179E-14 ) ) ;
#18181=AXIS2_PLACEMENT_3D ( 'NONE', #1889, #1495, #19181 ) ;
#18182=CYLINDRICAL_SURFACE ( 'NONE', #3378, 34.99999999999999289 ) ;
#18184=AXIS2_PLACEMENT_3D ( 'NONE', #1577, #6426, #12910 ) ;
#18189=AXIS2_PLACEMENT_3D ( 'NONE', #14099, #15672, #11195 ) ;
#18190=FACE_BOUND ( 'NONE', #7542, .T. ) ;
#18194=AXIS2_PLACEMENT_3D ( 'NONE', #6107, #9189, #10686 ) ;
#18197=CIRCLE ( 'NONE', #16175, 21.50000000000000000 ) ;
#18204=CARTESIAN_POINT ( 'NONE',  ( 21.50000000000000000, 2.632990618166809235E-15, -84.99999999999998579 ) ) ;
#18211=CARTESIAN_POINT ( 'NONE',  ( 31.01315681530222079, -111.3007080733049889, 79.47988500914458143 ) ) ;
#18215=EDGE_LOOP ( 'NONE', ( #5843, #17115, #8268, #15263 ) ) ;
#18230=LINE ( 'NONE', #11858, #15810 ) ;
#18232=ORIENTED_EDGE ( 'NONE', *, *, #7137, .F. ) ;
#18239=PLANE ( 'NONE',  #6467 ) ;
#18241=ORIENTED_EDGE ( 'NONE', *, *, #12825, .T. ) ;
#18244=SHAPE_REPRESENTATION_RELATIONSHIP ( 'NONE' , 'NONE' ,  #4392, #3656 ) ;
#18247=CARTESIAN_POINT ( 'NONE',  ( 37.20644374907093521, -120.3958613208574207, -85.16797049535011865 ) ) ;
#18255=CARTESIAN_POINT ( 'NONE',  ( -0.8281006575391447466, -21.49753944123813909, 70.58133206268971094 ) ) ;
#18257=VERTEX_POINT ( 'NONE', #4804 ) ;
#18263=EDGE_CURVE ( 'NONE', #19902, #13263, #17946, .T. ) ;
#18272=CARTESIAN_POINT ( 'NONE',  ( 30.00000000000000000, -99.99999999999998579, -54.09999999999998721 ) ) ;
#18275=CARTESIAN_POINT ( 'NONE',  ( -7.539743116613892404, -20.19060691129837792, -71.13878616268860355 ) ) ;
#18280=ADVANCED_FACE ( 'NONE', ( #6699 ), #1839, .F. ) ;
#18281=ORIENTED_EDGE ( 'NONE', *, *, #8747, .T. ) ;
#18283=AXIS2_PLACEMENT_3D ( 'NONE', #17637, #16248, #8094 ) ;
#18285=ORIENTED_EDGE ( 'NONE', *, *, #4033, .F. ) ;
#18286=DIRECTION ( 'NONE',  ( -1.000000000000000000, -0.000000000000000000, -0.000000000000000000 ) ) ;
#18294=ORIENTED_EDGE ( 'NONE', *, *, #7435, .F. ) ;
#18302=CARTESIAN_POINT ( 'NONE',  ( 30.00000000000000000, -170.8299878242309546, 15.48896927112552824 ) ) ;
#18304=ORIENTED_EDGE ( 'NONE', *, *, #1222, .T. ) ;
#18305=EDGE_CURVE ( 'NONE', #14577, #14343, #18150, .T. ) ;
#18306=CARTESIAN_POINT ( 'NONE',  ( 39.62815566457561545, -122.1058236485348374, 86.75687390987235403 ) ) ;
#18316=AXIS2_PLACEMENT_3D ( 'NONE', #11498, #1969, #14499 ) ;
#18319=CIRCLE ( 'NONE', #19011, 18.00000000000000000 ) ;
#18330=VECTOR ( 'NONE', #10098, 1000.000000000000000 ) ;
#18332=DIRECTION ( 'NONE',  ( 0.000000000000000000, 0.000000000000000000, 1.000000000000000000 ) ) ;
#18335=CIRCLE ( 'NONE', #6809, 11.50000000000000000 ) ;
#18336=ORIENTED_EDGE ( 'NONE', *, *, #5963, .F. ) ;
#18338=VERTEX_POINT ( 'NONE', #15386 ) ;
#18339=FACE_OUTER_BOUND ( 'NONE', #18945, .T. ) ;
#18344=SURFACE_SIDE_STYLE ('',( #13065 ) ) ;
#18348=CARTESIAN_POINT ( 'NONE',  ( 40.00000000000000711, -30.00000000000001421, -120.0000000000000142 ) ) ;
#18359=AXIS2_PLACEMENT_3D ( 'NONE', #8771, #13770, #5801 ) ;
#18368=EDGE_LOOP ( 'NONE', ( #12914, #3888, #17205, #4651 ) ) ;
#18371=LINE ( 'NONE', #13602, #9740 ) ;
#18378=AXIS2_PLACEMENT_3D ( 'NONE', #8000, #11176, #6401 ) ;
#18381=FACE_OUTER_BOUND ( 'NONE', #1547, .T. ) ;
#18383=CARTESIAN_POINT ( 'NONE',  ( 16.80529800326410239, -13.48305675317430108, -74.69048503828150842 ) ) ;
#18389=ORIENTED_EDGE ( 'NONE', *, *, #6647, .F. ) ;
#18395=FACE_OUTER_BOUND ( 'NONE', #8246, .T. ) ;
#18398=LINE ( 'NONE', #16913, #19525 ) ;
#18407=ADVANCED_FACE ( 'NONE', ( #15272 ), #2144, .F. ) ;
#18410=DIRECTION ( 'NONE',  ( 1.000000000000000000, 0.000000000000000000, 0.000000000000000000 ) ) ;
#18416=ORIENTED_EDGE ( 'NONE', *, *, #7537, .F. ) ;
#18423=CARTESIAN_POINT ( 'NONE',  ( 50.00000000000000000, 4.299168419249259188, 90.00000000000000000 ) ) ;
#18430=DIRECTION ( 'NONE',  ( 1.000000000000000000, 0.000000000000000000, 0.000000000000000000 ) ) ;
#18434=EDGE_CURVE ( 'NONE', #10469, #14887, #10305, .T. ) ;
#18458=CARTESIAN_POINT ( 'NONE',  ( 30.32391323356592139, -108.7007521017901439, -78.47408402981700704 ) ) ;
#18461=DIRECTION ( 'NONE',  ( -0.000000000000000000, 0.000000000000000000, -1.000000000000000000 ) ) ;
#18468=CARTESIAN_POINT ( 'NONE',  ( -10.25561400234659004, -18.90011081285701877, 71.73813932909899904 ) ) ;
#18472=AXIS2_PLACEMENT_3D ( 'NONE', #18671, #2568, #7427 ) ;
#18474=CARTESIAN_POINT ( 'NONE',  ( 28.13963350654227824, -26.35784117651622793, -130.0000000000000000 ) ) ;
#18477=CARTESIAN_POINT ( 'NONE',  ( 22.70866746290765903, -3.649167310370807105, -90.00000000000000000 ) ) ;
#18485=VERTEX_POINT ( 'NONE', #16968 ) ;
#18487=VECTOR ( 'NONE', #11764, 1000.000000000000000 ) ;
#18488=CARTESIAN_POINT ( 'NONE',  ( 30.00000000000000000, -99.99999999999998579, -54.09999999999999432 ) ) ;
#18491=CARTESIAN_POINT ( 'NONE',  ( -14.94551481348181809, -15.47228562136405827, -73.52041642655927944 ) ) ;
#18493=EDGE_CURVE ( 'NONE', #1745, #8829, #13390, .T. ) ;
#18509=ORIENTED_EDGE ( 'NONE', *, *, #1996, .F. ) ;
#18518=CARTESIAN_POINT ( 'NONE',  ( -5.705422232504516522, -20.77800788743411076, 76.38232661121730871 ) ) ;
#18524=CARTESIAN_POINT ( 'NONE',  ( 29.99999999999999645, -105.9493285778136595, 77.66804255791004152 ) ) ;
#18526=VECTOR ( 'NONE', #11439, 1000.000000000000000 ) ;
#18529=CARTESIAN_POINT ( 'NONE',  ( 7.582106015220150930, -21.76672924613218996, -75.91315008488570015 ) ) ;
#18530=VERTEX_POINT ( 'NONE', #14124 ) ;
#18531=CARTESIAN_POINT ( 'NONE',  ( 0.000000000000000000, 0.000000000000000000, 81.99999999999998579 ) ) ;
#18534=EDGE_CURVE ( 'NONE', #834, #9768, #2672, .T. ) ;
#18538=CIRCLE ( 'NONE', #9404, 5.000000000000004441 ) ;
#18547=DIRECTION ( 'NONE',  ( 1.000000000000000000, 0.000000000000000000, 0.000000000000000000 ) ) ;
#18556=ORIENTED_EDGE ( 'NONE', *, *, #20607, .T. ) ;
#18563=ORIENTED_EDGE ( 'NONE', *, *, #4958, .F. ) ;
#18576=ORIENTED_EDGE ( 'NONE', *, *, #10308, .T. ) ;
#18580=CARTESIAN_POINT ( 'NONE',  ( -13.32881486730457610, -16.88549087568889107, 72.74798471664088595 ) ) ;
#18592=DIRECTION ( 'NONE',  ( -0.000000000000000000, -0.000000000000000000, 1.000000000000000000 ) ) ;
#18594=ORIENTED_EDGE ( 'NONE', *, *, #13376, .T. ) ;
#18598=CARTESIAN_POINT ( 'NONE',  ( 20.76542986210400343, -5.602711969362187183, -80.65560201174187682 ) ) ;
#18602=DIRECTION ( 'NONE',  ( 1.000000000000000000, 0.000000000000000000, -0.000000000000000000 ) ) ;
#18604=CARTESIAN_POINT ( 'NONE',  ( 50.00000000000000000, -1.326995226329893862, 84.99999999999998579 ) ) ;
#18605=EDGE_LOOP ( 'NONE', ( #2662, #12778 ) ) ;
#18608=FACE_OUTER_BOUND ( 'NONE', #13206, .T. ) ;
#18609=APPLICATION_CONTEXT ( 'automotive_design' ) ;
#18610=DIRECTION ( 'NONE',  ( -1.000000000000000000, 0.000000000000000000, 0.000000000000000000 ) ) ;
#18615=VERTEX_POINT ( 'NONE', #1307 ) ;
#18622=CARTESIAN_POINT ( 'NONE',  ( 35.37092464391603386, -118.6634975751123591, 83.76198506216627493 ) ) ;
#18624=EDGE_LOOP ( 'NONE', ( #9326, #20070, #8558, #14816 ) ) ;
#18625=CARTESIAN_POINT ( 'NONE',  ( -0.7189812636139246704, -23.00150371214196809, -75.37276332846732885 ) ) ;
#18635=CARTESIAN_POINT ( 'NONE',  ( 30.00000000000000711, -30.00000000000001421, -130.0000000000000000 ) ) ;
#18642=ADVANCED_FACE ( 'NONE', ( #14018, #12423 ), #9238, .F. ) ;
#18646=ORIENTED_EDGE ( 'NONE', *, *, #7181, .F. ) ;
#18649=DIRECTION ( 'NONE',  ( 0.000000000000000000, 0.000000000000000000, -1.000000000000000000 ) ) ;
#18650=ORIENTED_EDGE ( 'NONE', *, *, #11943, .F. ) ;
#18655=CARTESIAN_POINT ( 'NONE',  ( 37.35049175653090714, -20.28192400168857645, -71.09734905643766467 ) ) ;
#18656=VERTEX_POINT ( 'NONE', #9547 ) ;
#18658=EDGE_LOOP ( 'NONE', ( #6234, #11233, #14751, #15163 ) ) ;
#18666=EDGE_CURVE ( 'NONE', #5687, #20286, #14843, .T. ) ;
#18667=CARTESIAN_POINT ( 'NONE',  ( 10.00000000000000178, -160.0000000000000000, -73.20000000000000284 ) ) ;
#18671=CARTESIAN_POINT ( 'NONE',  ( 0.000000000000000000, 0.000000000000000000, 68.00000000000000000 ) ) ;
#18673=FACE_OUTER_BOUND ( 'NONE', #5242, .T. ) ;
#18675=EDGE_CURVE ( 'NONE', #7631, #2747, #17827, .T. ) ;
#18677=CARTESIAN_POINT ( 'NONE',  ( -9.249412617561585392, -19.41235462500713993, 71.49717528132291022 ) ) ;
#18682=VERTEX_POINT ( 'NONE', #3192 ) ;
#18683=DIRECTION ( 'NONE',  ( 0.000000000000000000, -1.000000000000000000, -8.673617379884035472E-17 ) ) ;
#18686=VERTEX_POINT ( 'NONE', #19502 ) ;
#18687=CYLINDRICAL_SURFACE ( 'NONE', #15758, 5.000000000000004441 ) ;
#18688=VECTOR ( 'NONE', #9989, 1000.000000000000000 ) ;
#18690=EDGE_CURVE ( 'NONE', #4727, #8495, #3386, .T. ) ;
#18700=CYLINDRICAL_SURFACE ( 'NONE', #5084, 3.199999999999994404 ) ;
#18701=ORIENTED_EDGE ( 'NONE', *, *, #152, .F. ) ;
#18709=DIRECTION ( 'NONE',  ( 0.000000000000000000, 0.000000000000000000, -1.000000000000000000 ) ) ;
#18717=CIRCLE ( 'NONE', #2133, 39.99999999999999289 ) ;
#18724=EDGE_LOOP ( 'NONE', ( #14392, #12787, #14696, #8732 ) ) ;
#18725=DIRECTION ( 'NONE',  ( -1.000000000000000000, 0.000000000000000000, 0.000000000000000000 ) ) ;
#18728=CARTESIAN_POINT ( 'NONE',  ( -20.21355047154532159, -7.393864663665485004, 85.82585403120822320 ) ) ;
#18734=VECTOR ( 'NONE', #1847, 1000.000000000000000 ) ;
#18740=ORIENTED_EDGE ( 'NONE', *, *, #5387, .F. ) ;
#18741=CARTESIAN_POINT ( 'NONE',  ( 16.48273624093881651, -16.04508369211728436, -78.99984814018115742 ) ) ;
#18745=VERTEX_POINT ( 'NONE', #7 ) ;
#18748=CYLINDRICAL_SURFACE ( 'NONE', #2279, 14.49999999999999467 ) ;
#18750=VECTOR ( 'NONE', #16551, 1000.000000000000000 ) ;
#18751=DIRECTION ( 'NONE',  ( 1.000000000000000000, 0.000000000000000000, 0.000000000000000000 ) ) ;
#18752=CARTESIAN_POINT ( 'NONE',  ( 40.00000000000000711, -30.00000000000001421, -130.0000000000000000 ) ) ;
#18753=DIRECTION ( 'NONE',  ( 0.000000000000000000, 0.000000000000000000, -1.000000000000000000 ) ) ;
#18768=DIRECTION ( 'NONE',  ( 1.000000000000000000, -0.000000000000000000, -0.000000000000000000 ) ) ;
#18769=ORIENTED_EDGE ( 'NONE', *, *, #11782, .T. ) ;
#18772=CIRCLE ( 'NONE', #19424, 10.00000000000000178 ) ;
#18773=DIRECTION ( 'NONE',  ( 0.000000000000000000, 0.000000000000000000, -1.000000000000000000 ) ) ;
#18775=ORIENTED_EDGE ( 'NONE', *, *, #7732, .F. ) ;
#18781=VECTOR ( 'NONE', #14131, 1000.000000000000000 ) ;
#18785=FACE_OUTER_BOUND ( 'NONE', #20420, .T. ) ;
#18786=ORIENTED_EDGE ( 'NONE', *, *, #20751, .F. ) ;
#18799=CARTESIAN_POINT ( 'NONE',  ( 10.00000000000000178, -164.9999999999999716, 73.20000000000000284 ) ) ;
#18802=CARTESIAN_POINT ( 'NONE',  ( 47.99913302141637672, -4.465704580667244628, 88.98724172780553943 ) ) ;
#18821=CARTESIAN_POINT ( 'NONE',  ( 30.00000000000001066, 39.99999999999998579, -120.0000000000000142 ) ) ;
#18836=ORIENTED_EDGE ( 'NONE', *, *, #8071, .F. ) ;
#18845=DIRECTION ( 'NONE',  ( 0.000000000000000000, 0.000000000000000000, -1.000000000000000000 ) ) ;
#18848=CARTESIAN_POINT ( 'NONE',  ( 20.64343997858507862, -10.14597586228817860, -83.32269133937376182 ) ) ;
#18849=DIRECTION ( 'NONE',  ( 0.000000000000000000, 0.000000000000000000, -1.000000000000000000 ) ) ;
#18857=AXIS2_PLACEMENT_3D ( 'NONE', #101, #8455, #19595 ) ;
#18859=CARTESIAN_POINT ( 'NONE',  ( 30.00000000000000000, -99.99999999999998579, 49.89999999999999858 ) ) ;
#18862=AXIS2_PLACEMENT_3D ( 'NONE', #1149, #15541, #7599 ) ;
#18875=CARTESIAN_POINT ( 'NONE',  ( 50.00000000000000000, -160.0000000000000000, -79.59486983196737242 ) ) ;
#18877=CARTESIAN_POINT ( 'NONE',  ( 30.00000000000000000, -39.99999999999999289, 52.00000000000000000 ) ) ;
#18880=DIRECTION ( 'NONE',  ( 1.000000000000000000, 0.000000000000000000, 0.000000000000000000 ) ) ;
#18889=EDGE_CURVE ( 'NONE', #19472, #16235, #18230, .T. ) ;
#18891=AXIS2_PLACEMENT_3D ( 'NONE', #19856, #11593, #14987 ) ;
#18892=CARTESIAN_POINT ( 'NONE',  ( 24.99999999999999645, -99.99999999999998579, 49.89999999999999858 ) ) ;
#18902=CARTESIAN_POINT ( 'NONE',  ( 40.00000000000000711, -40.00000000000001421, -120.0000000000000142 ) ) ;
#18903=ORIENTED_EDGE ( 'NONE', *, *, #152, .T. ) ;
#18919=ADVANCED_FACE ( 'NONE', ( #20232 ), #8678, .F. ) ;
#18926=LINE ( 'NONE', #14257, #17745 ) ;
#18931=ORIENTED_EDGE ( 'NONE', *, *, #8561, .T. ) ;
#18936=VERTEX_POINT ( 'NONE', #734 ) ;
#18939=CARTESIAN_POINT ( 'NONE',  ( -30.00000000000000000, 40.00000000000000000, -120.0000000000000142 ) ) ;
#18942=EDGE_CURVE ( 'NONE', #10714, #6265, #19877, .T. ) ;
#18945=EDGE_LOOP ( 'NONE', ( #16107, #18646 ) ) ;
#18950=CARTESIAN_POINT ( 'NONE',  ( 11.67222246750216463, -19.83243759501799630, -76.85199795501601727 ) ) ;
#18956=DIRECTION ( 'NONE',  ( 0.000000000000000000, 0.000000000000000000, -1.000000000000000000 ) ) ;
#18961=ADVANCED_FACE ( 'NONE', ( #20553 ), #3241, .F. ) ;
#18965=CARTESIAN_POINT ( 'NONE',  ( 50.00000000000000000, -164.9999999999999716, -90.00000000000001421 ) ) ;
#18967=EDGE_CURVE ( 'NONE', #14001, #12159, #15473, .T. ) ;
#18968=AXIS2_PLACEMENT_3D ( 'NONE', #5216, #5513, #13490 ) ;
#18971=DIRECTION ( 'NONE',  ( 1.000000000000000000, -1.734723475976806848E-16, -0.000000000000000000 ) ) ;
#18977=CARTESIAN_POINT ( 'NONE',  ( 34.40748350626766694, -26.49925741089600706, -73.93400743789861451 ) ) ;
#18981=ORIENTED_EDGE ( 'NONE', *, *, #18023, .F. ) ;
#18987=VECTOR ( 'NONE', #1964, 1000.000000000000000 ) ;
#18989=CARTESIAN_POINT ( 'NONE',  ( 18.00000000000000000, 0.000000000000000000, -130.0000000000000000 ) ) ;
#18993=ORIENTED_EDGE ( 'NONE', *, *, #8798, .T. ) ;
#18995=CARTESIAN_POINT ( 'NONE',  ( 30.00000000000000000, 4.299168419249259188, 89.99999999999998579 ) ) ;
#18999=ORIENTED_EDGE ( 'NONE', *, *, #15288, .T. ) ;
#19004=ORIENTED_EDGE ( 'NONE', *, *, #3690, .F. ) ;
#19011=AXIS2_PLACEMENT_3D ( 'NONE', #9222, #12731, #12407 ) ;
#19017=CARTESIAN_POINT ( 'NONE',  ( 11.50000000000000000, 1.408343819019456176E-15, -68.00000000000000000 ) ) ;
#19020=B_SPLINE_CURVE_WITH_KNOTS ( 'NONE', 3,
 ( #4081, #12047, #5779, #18728, #13960, #12255, #12371, #10781, #5678, #10679, #13640, #2622, #12150, #20413, #20088, #19980, #10564, #17028, #17244, #5462, #5567, #2516, #18518, #4409, #9602, #2823, #3135, #19044, #12693, #1355, #7799, #6412, #14274, #15644, #20721, #15862, #1252, #4519, #4831, #7706, #9181, #6209, #16072, #1564, #17460, #9496, #19151, #20621, #12475, #6097, #4728, #9403, #10984, #12575, #4624, #19346 ),
 .UNSPECIFIED., .F., .F.,
 ( 4, 2, 2, 2, 2, 2, 2, 2, 2, 2, 2, 2, 2, 2, 2, 2, 2, 2, 2, 2, 2, 2, 2, 2, 2, 2, 2, 4 ),
 ( 7.372574772901430151E-18, 0.004247431497134123227, 0.008494862994268239514, 0.01061857874283529332, 0.01168043661711882369, 0.01274229449140235233, 0.01698972598853643393, 0.01911344173710348426, 0.02123715748567053460, 0.02336087323423758841, 0.02548458898280463528, 0.02973202047993872901, 0.03185573622850577935, 0.03397945197707283316, 0.03822688347420693383, 0.04035059922277398070, 0.04247431497134102757, 0.04459803071990808832, 0.04565988859419161522, 0.04672174646847514212, 0.05096917796560924280, 0.05203103583989275582, 0.05309289371417626191, 0.05521660946274327408, 0.05734032521131028626, 0.05946404095987729843, 0.06371147245701133666, 0.06795890395414536100 ),
 .UNSPECIFIED. ) ;
#19024=AXIS2_PLACEMENT_3D ( 'NONE', #4537, #1049, #18956 ) ;
#19028=CARTESIAN_POINT ( 'NONE',  ( -22.96694501150314238, -24.74873734152930993, -130.0000000000000000 ) ) ;
#19030=AXIS2_PLACEMENT_3D ( 'NONE', #17704, #19382, #14620 ) ;
#19031=CIRCLE ( 'NONE', #20020, 2.099999999999997868 ) ;
#19039=EDGE_LOOP ( 'NONE', ( #13548, #20890, #9329, #19344 ) ) ;
#19044=CARTESIAN_POINT ( 'NONE',  ( 1.400806052880371855, -21.50201457020015283, 76.03989839961199948 ) ) ;
#19061=EDGE_CURVE ( 'NONE', #10075, #10995, #6338, .T. ) ;
#19065=VECTOR ( 'NONE', #11191, 1000.000000000000000 ) ;
#19070=CIRCLE ( 'NONE', #5177, 80.00000000000000000 ) ;
#19074=DIRECTION ( 'NONE',  ( 0.000000000000000000, -1.000000000000000000, 0.000000000000000000 ) ) ;
#19088=CARTESIAN_POINT ( 'NONE',  ( 29.99999999999999645, -106.8586209199411314, -72.71093006432944605 ) ) ;
#19089=AXIS2_PLACEMENT_3D ( 'NONE', #14044, #11162, #15927 ) ;
#19091=ADVANCED_FACE ( 'NONE', ( #4833 ), #17776, .T. ) ;
#19104=AXIS2_PLACEMENT_3D ( 'NONE', #3018, #19236, #10859 ) ;
#19113=VERTEX_POINT ( 'NONE', #5811 ) ;
#19118=ORIENTED_EDGE ( 'NONE', *, *, #15552, .F. ) ;
#19119=LINE ( 'NONE', #17312, #5591 ) ;
#19126=EDGE_CURVE ( 'NONE', #1656, #3436, #3949, .T. ) ;
#19138=ORIENTED_EDGE ( 'NONE', *, *, #15798, .F. ) ;
#19151=CARTESIAN_POINT ( 'NONE',  ( 17.18811727938071598, -12.93019132815889627, 81.11311984140925802 ) ) ;
#19156=LINE ( 'NONE', #19459, #6337 ) ;
#19157=DIRECTION ( 'NONE',  ( -1.000000000000000000, 0.000000000000000000, 0.000000000000000000 ) ) ;
#19158=ORIENTED_EDGE ( 'NONE', *, *, #11143, .F. ) ;
#19159=CARTESIAN_POINT ( 'NONE',  ( -20.49352359574021065, -10.45859730899524820, -83.05345869059719632 ) ) ;
#19180=CARTESIAN_POINT ( 'NONE',  ( 30.00000000000000000, -85.00000000000000000, -1.040949779275250179E-14 ) ) ;
#19181=DIRECTION ( 'NONE',  ( -1.000000000000000000, 1.734723475976806848E-16, 0.000000000000000000 ) ) ;
#19205=ORIENTED_EDGE ( 'NONE', *, *, #3654, .F. ) ;
#19210=DIRECTION ( 'NONE',  ( 1.000000000000000000, 0.000000000000000000, 0.000000000000000000 ) ) ;
#19211=VERTEX_POINT ( 'NONE', #13311 ) ;
#19219=CIRCLE ( 'NONE', #6019, 80.00000000000000000 ) ;
#19223=CARTESIAN_POINT ( 'NONE',  ( 40.00000000000000711, -40.00000000000001421, -130.0000000000000000 ) ) ;
#19225=ORIENTED_EDGE ( 'NONE', *, *, #803, .F. ) ;
#19232=ORIENTED_EDGE ( 'NONE', *, *, #2610, .T. ) ;
#19234=EDGE_CURVE ( 'NONE', #5499, #9196, #10356, .T. ) ;
#19236=DIRECTION ( 'NONE',  ( 0.000000000000000000, -1.000000000000000000, 0.000000000000000000 ) ) ;
#19241=ORIENTED_EDGE ( 'NONE', *, *, #5461, .F. ) ;
#19246=LINE ( 'NONE', #1664, #18109 ) ;
#19257=CARTESIAN_POINT ( 'NONE',  ( -17.19777750590179366, -15.33753975069672748, -79.43571204742693226 ) ) ;
#19264=CARTESIAN_POINT ( 'NONE',  ( -30.00000000000000000, -85.00000000000000000, 8.999999999999984013 ) ) ;
#19267=DIRECTION ( 'NONE',  ( 0.000000000000000000, -1.000000000000000000, 0.000000000000000000 ) ) ;
#19270=DIRECTION ( 'NONE',  ( 1.000000000000000000, 0.000000000000000000, 0.000000000000000000 ) ) ;
#19274=CARTESIAN_POINT ( 'NONE',  ( 50.00000000000000000, -164.9999999999999716, -75.59990929030051632 ) ) ;
#19277=ORIENTED_EDGE ( 'NONE', *, *, #6020, .F. ) ;
#19281=EDGE_LOOP ( 'NONE', ( #6960, #13424, #8831, #12361 ) ) ;
#19285=DIRECTION ( 'NONE',  ( -1.000000000000000000, 0.000000000000000000, 0.000000000000000000 ) ) ;
#19289=DIRECTION ( 'NONE',  ( 1.000000000000000000, -0.000000000000000000, -0.000000000000000000 ) ) ;
#19292=ADVANCED_FACE ( 'NONE', ( #8216 ), #3745, .F. ) ;
#19294=LINE ( 'NONE', #8375, #12611 ) ;
#19303=CARTESIAN_POINT ( 'NONE',  ( 30.47229197614141682, -42.00316239176417099, 71.34654888422416263 ) ) ;
#19305=VECTOR ( 'NONE', #2962, 1000.000000000000000 ) ;
#19314=EDGE_LOOP ( 'NONE', ( #13301, #6937, #18769, #8164, #621, #7737, #15409, #10911, #793 ) ) ;
#19342=EDGE_CURVE ( 'NONE', #8829, #10337, #20166, .T. ) ;
#19344=ORIENTED_EDGE ( 'NONE', *, *, #16642, .T. ) ;
#19346=CARTESIAN_POINT ( 'NONE',  ( 21.18805271706017024, -3.649167310370820871, 90.00000000000000000 ) ) ;
#19347=AXIS2_PLACEMENT_3D ( 'NONE', #10934, #5842, #15811 ) ;
#19357=ADVANCED_FACE ( 'NONE', ( #15309 ), #15206, .T. ) ;
#19358=CARTESIAN_POINT ( 'NONE',  ( 30.00000000000000000, -42.57363661491096707, -66.38288848018790134 ) ) ;
#19371=CARTESIAN_POINT ( 'NONE',  ( 23.13963350654227824, -26.35784117651622793, -120.0000000000000142 ) ) ;
#19372=VECTOR ( 'NONE', #1163, 1000.000000000000000 ) ;
#19377=CARTESIAN_POINT ( 'NONE',  ( 38.21638006031223966, -18.69091178866597147, 71.83091255860625779 ) ) ;
#19382=DIRECTION ( 'NONE',  ( -0.000000000000000000, -1.000000000000000000, -0.000000000000000000 ) ) ;
#19390=AXIS2_PLACEMENT_3D ( 'NONE', #8850, #10776, #12143 ) ;
#19395=EDGE_CURVE ( 'NONE', #13475, #16876, #15830, .T. ) ;
#19396=DIRECTION ( 'NONE',  ( 0.000000000000000000, 0.000000000000000000, -1.000000000000000000 ) ) ;
#19401=EDGE_LOOP ( 'NONE', ( #11811, #2311, #3123, #2906 ) ) ;
#19405=FACE_OUTER_BOUND ( 'NONE', #8695, .T. ) ;
#19406=AXIS2_PLACEMENT_3D ( 'NONE', #8410, #359, #6925 ) ;
#19408=VECTOR ( 'NONE', #3331, 1000.000000000000000 ) ;
#19416=VECTOR ( 'NONE', #8096, 1000.000000000000000 ) ;
#19424=AXIS2_PLACEMENT_3D ( 'NONE', #2914, #12458, #12675 ) ;
#19428=CARTESIAN_POINT ( 'NONE',  ( 23.00000000000000000, 0.000000000000000000, -120.0000000000000142 ) ) ;
#19429=ORIENTED_EDGE ( 'NONE', *, *, #1946, .F. ) ;
#19430=FACE_OUTER_BOUND ( 'NONE', #14363, .T. ) ;
#19433=ORIENTED_EDGE ( 'NONE', *, *, #3208, .T. ) ;
#19436=EDGE_LOOP ( 'NONE', ( #5137, #9058 ) ) ;
#19439=EDGE_LOOP ( 'NONE', ( #17735, #1606 ) ) ;
#19451=ADVANCED_FACE ( 'NONE', ( #5549 ), #2491, .F. ) ;
#19456=ADVANCED_FACE ( 'NONE', ( #5759 ), #4179, .T. ) ;
#19457=VERTEX_POINT ( 'NONE', #5879 ) ;
#19459=CARTESIAN_POINT ( 'NONE',  ( 30.00000000000000000, -85.00000000000000000, -45.00000000000000711 ) ) ;
#19460=DIRECTION ( 'NONE',  ( 0.000000000000000000, 0.000000000000000000, -1.000000000000000000 ) ) ;
#19466=ORIENTED_EDGE ( 'NONE', *, *, #14429, .F. ) ;
#19467=CARTESIAN_POINT ( 'NONE',  ( 50.00000000000000000, 36.35083268962915781, -50.00000000000000000 ) ) ;
#19472=VERTEX_POINT ( 'NONE', #12784 ) ;
#19474=CARTESIAN_POINT ( 'NONE',  ( 0.000000000000000000, 0.000000000000000000, 0.000000000000000000 ) ) ;
#19477=CIRCLE ( 'NONE', #18137, 80.00000000000000000 ) ;
#19479=CIRCLE ( 'NONE', #5617, 2.099999999999990763 ) ;
#19488=CARTESIAN_POINT ( 'NONE',  ( 44.32616946416951720, -9.742112414153938360, -83.66536569035999094 ) ) ;
#19490=ORIENTED_EDGE ( 'NONE', *, *, #19974, .F. ) ;
#19492=CARTESIAN_POINT ( 'NONE',  ( 49.19234958605026264, -1.326995226329893862, 84.99999999999998579 ) ) ;
#19498=LINE ( 'NONE', #4881, #17664 ) ;
#19502=CARTESIAN_POINT ( 'NONE',  ( 23.00000000000000000, 0.000000000000000000, -90.00000000000000000 ) ) ;
#19511=VECTOR ( 'NONE', #12879, 1000.000000000000000 ) ;
#19512=EDGE_LOOP ( 'NONE', ( #16718, #2978 ) ) ;
#19513=VECTOR ( 'NONE', #686, 1000.000000000000000 ) ;
#19514=CYLINDRICAL_SURFACE ( 'NONE', #4072, 205.0000000000000284 ) ;
#19515=CARTESIAN_POINT ( 'NONE',  ( 45.22159793441011999, -8.673994507468384185, 84.62946326583127643 ) ) ;
#19517=EDGE_LOOP ( 'NONE', ( #4873, #3989 ) ) ;
#19525=VECTOR ( 'NONE', #18610, 1000.000000000000000 ) ;
#19538=CARTESIAN_POINT ( 'NONE',  ( 50.00000000000000000, -49.99999999999999289, -71.93747284969079203 ) ) ;
#19540=ORIENTED_EDGE ( 'NONE', *, *, #1348, .T. ) ;
#19541=LINE ( 'NONE', #8103, #18734 ) ;
#19544=CIRCLE ( 'NONE', #11094, 11.49999999999999645 ) ;
#19545=ORIENTED_EDGE ( 'NONE', *, *, #11782, .F. ) ;
#19546=AXIS2_PLACEMENT_3D ( 'NONE', #1211, #11053, #4693 ) ;
#19553=VERTEX_POINT ( 'NONE', #15736 ) ;
#19555=CIRCLE ( 'NONE', #3960, 80.00000000000000000 ) ;
#19561=CARTESIAN_POINT ( 'NONE',  ( -30.00000000000000000, -30.00000000000000000, -120.0000000000000142 ) ) ;
#19571=DIRECTION ( 'NONE',  ( 0.7071067811865445751, 0.4413865154835797666, -0.5524291302504493739 ) ) ;
#19573=EDGE_CURVE ( 'NONE', #4727, #1571, #10377, .T. ) ;
#19577=DIRECTION ( 'NONE',  ( 0.000000000000000000, 0.000000000000000000, -1.000000000000000000 ) ) ;
#19581=EDGE_CURVE ( 'NONE', #10704, #1189, #15937, .T. ) ;
#19583=EDGE_LOOP ( 'NONE', ( #18285, #14085, #14022, #17034, #7021, #12492 ) ) ;
#19585=DIRECTION ( 'NONE',  ( 0.000000000000000000, 0.000000000000000000, 1.000000000000000000 ) ) ;
#19586=CARTESIAN_POINT ( 'NONE',  ( 33.92785236135936344, -27.95564457753036436, 68.35308193655099274 ) ) ;
#19590=DIRECTION ( 'NONE',  ( -1.000000000000000000, -0.000000000000000000, -0.000000000000000000 ) ) ;
#19591=CARTESIAN_POINT ( 'NONE',  ( -30.00000000000000000, -3.649167310370807105, -90.00000000000000000 ) ) ;
#19594=ORIENTED_EDGE ( 'NONE', *, *, #9539, .T. ) ;
#19595=DIRECTION ( 'NONE',  ( 0.000000000000000000, 0.000000000000000000, -1.000000000000000000 ) ) ;
#19596=ADVANCED_FACE ( 'NONE', ( #1545 ), #1337, .T. ) ;
#19597=CARTESIAN_POINT ( 'NONE',  ( 30.00000000000000000, -99.99999999999998579, 54.09999999999998721 ) ) ;
#19604=DIRECTION ( 'NONE',  ( 0.000000000000000000, -0.000000000000000000, 1.000000000000000000 ) ) ;
#19605=CARTESIAN_POINT ( 'NONE',  ( 30.00000000000000000, -122.0000000000000000, -6.368163355566234804E-15 ) ) ;
#19607=LINE ( 'NONE', #9961, #2444 ) ;
#19609=LINE ( 'NONE', #8271, #17763 ) ;
#19610=ORIENTED_EDGE ( 'NONE', *, *, #7411, .T. ) ;
#19615=VERTEX_POINT ( 'NONE', #7997 ) ;
#19616=ORIENTED_EDGE ( 'NONE', *, *, #7060, .F. ) ;
#19620=CARTESIAN_POINT ( 'NONE',  ( 0.000000000000000000, 0.000000000000000000, -68.00000000000000000 ) ) ;
#19632=DIRECTION ( 'NONE',  ( -1.000000000000000000, 0.000000000000000000, 0.000000000000000000 ) ) ;
#19637=CARTESIAN_POINT ( 'NONE',  ( 50.00000000000000000, -164.9999999999999716, 90.00000000000001421 ) ) ;
#19641=DIRECTION ( 'NONE',  ( 1.000000000000000000, 0.000000000000000000, 0.000000000000000000 ) ) ;
#19646=CYLINDRICAL_SURFACE ( 'NONE', #6932, 34.99999999999999289 ) ;
#19648=VERTEX_POINT ( 'NONE', #12457 ) ;
#19654=DIRECTION ( 'NONE',  ( -1.000000000000000000, 0.000000000000000000, 0.000000000000000000 ) ) ;
#19655=VERTEX_POINT ( 'NONE', #3626 ) ;
#19656=PLANE ( 'NONE',  #15126 ) ;
#19669=CIRCLE ( 'NONE', #17986, 5.000000000000004441 ) ;
#19672=AXIS2_PLACEMENT_3D ( 'NONE', #2203, #6963, #3778 ) ;
#19679=CARTESIAN_POINT ( 'NONE',  ( -24.99999999999999289, -160.0000000000000000, 0.000000000000000000 ) ) ;
#19692=CARTESIAN_POINT ( 'NONE',  ( -8.500000000000000000, 0.000000000000000000, -90.00000000000000000 ) ) ;
#19710=DIRECTION ( 'NONE',  ( -1.000000000000000000, 0.000000000000000000, 0.000000000000000000 ) ) ;
#19712=VERTEX_POINT ( 'NONE', #18056 ) ;
#19729=CARTESIAN_POINT ( 'NONE',  ( 30.00000000000000711, -40.00000000000001421, -120.0000000000000142 ) ) ;
#19730=VECTOR ( 'NONE', #17284, 1000.000000000000000 ) ;
#19733=FACE_OUTER_BOUND ( 'NONE', #903, .T. ) ;
#19740=PLANE ( 'NONE',  #4114 ) ;
#19741=EDGE_LOOP ( 'NONE', ( #17099, #6130, #19225, #4199 ) ) ;
#19750=VECTOR ( 'NONE', #1705, 1000.000000000000000 ) ;
#19759=ORIENTED_EDGE ( 'NONE', *, *, #4275, .F. ) ;
#19762=ORIENTED_EDGE ( 'NONE', *, *, #9696, .F. ) ;
#19769=CARTESIAN_POINT ( 'NONE',  ( 45.76122707727121508, -127.3290820621008947, -85.00000000000000000 ) ) ;
#19771=DIRECTION ( 'NONE',  ( 1.000000000000000000, 0.000000000000000000, 0.000000000000000000 ) ) ;
#19774=CARTESIAN_POINT ( 'NONE',  ( -18.00000000000000000, 2.204364238465235428E-15, -130.0000000000000000 ) ) ;
#19781=AXIS2_PLACEMENT_3D ( 'NONE', #6911, #10199, #12001 ) ;
#19789=EDGE_LOOP ( 'NONE', ( #19158, #8498, #15219, #6551 ) ) ;
#19799=CARTESIAN_POINT ( 'NONE',  ( 50.00000000000000000, 36.35083268962915781, -50.00000000000000000 ) ) ;
#19805=EDGE_CURVE ( 'NONE', #2608, #5687, #20875, .T. ) ;
#19811=CARTESIAN_POINT ( 'NONE',  ( 0.000000000000000000, 0.000000000000000000, -120.0000000000000142 ) ) ;
#19821=FACE_OUTER_BOUND ( 'NONE', #10757, .T. ) ;
#19823=CIRCLE ( 'NONE', #10005, 34.99999999999999289 ) ;
#19824=ORIENTED_EDGE ( 'NONE', *, *, #6598, .F. ) ;
#19827=AXIS2_PLACEMENT_3D ( 'NONE', #7753, #7533, #10828 ) ;
#19834=EDGE_CURVE ( 'NONE', #2130, #9768, #16472, .T. ) ;
#19845=CARTESIAN_POINT ( 'NONE',  ( -18.69829135368511075, -10.63264222386861135, 76.60301815488043076 ) ) ;
#19846=VERTEX_POINT ( 'NONE', #15993 ) ;
#19852=VERTEX_POINT ( 'NONE', #6654 ) ;
#19856=CARTESIAN_POINT ( 'NONE',  ( 30.00000000000000000, -99.99999999999998579, 52.00000000000000000 ) ) ;
#19858=CARTESIAN_POINT ( 'NONE',  ( 24.99999999999999645, -39.99999999999999289, 52.00000000000000000 ) ) ;
#19864=DIRECTION ( 'NONE',  ( 0.000000000000000000, 0.000000000000000000, 1.000000000000000000 ) ) ;
#19865=ADVANCED_FACE ( 'NONE', ( #18104 ), #11222, .T. ) ;
#19873=DIRECTION ( 'NONE',  ( -1.000000000000000000, 0.000000000000000000, 0.000000000000000000 ) ) ;
#19874=FACE_OUTER_BOUND ( 'NONE', #10197, .T. ) ;
#19876=ORIENTED_EDGE ( 'NONE', *, *, #5169, .T. ) ;
#19877=CIRCLE ( 'NONE', #4649, 5.000000000000004441 ) ;
#19878=CARTESIAN_POINT ( 'NONE',  ( 50.00000000000000000, -160.0000000000000000, 0.000000000000000000 ) ) ;
#19885=DIRECTION ( 'NONE',  ( 1.000000000000000000, -0.000000000000000000, -0.000000000000000000 ) ) ;
#19896=DIRECTION ( 'NONE',  ( -1.000000000000000000, 0.000000000000000000, 0.000000000000000000 ) ) ;
#19902=VERTEX_POINT ( 'NONE', #3366 ) ;
#19903=ORIENTED_EDGE ( 'NONE', *, *, #2295, .F. ) ;
#19904=DIRECTION ( 'NONE',  ( 0.000000000000000000, -0.7812527682501556603, 0.6242147964454771714 ) ) ;
#19913=ORIENTED_EDGE ( 'NONE', *, *, #10375, .T. ) ;
#19914=EDGE_CURVE ( 'NONE', #14529, #3964, #20527, .T. ) ;
#19915=CARTESIAN_POINT ( 'NONE',  ( 21.45900938229203447, -1.326995226329880762, -84.99999999999998579 ) ) ;
#19936=CARTESIAN_POINT ( 'NONE',  ( 28.06187315134367566, -160.0000000000000000, -51.51416696573247833 ) ) ;
#19939=CARTESIAN_POINT ( 'NONE',  ( 4.119954785698633160, -21.10500016855061389, 70.74589478160184797 ) ) ;
#19941=CARTESIAN_POINT ( 'NONE',  ( -18.00000000000000000, 2.204364238465235428E-15, -90.00000000000000000 ) ) ;
#19959=CARTESIAN_POINT ( 'NONE',  ( -3.108800563652526439, -21.28778730843814415, -70.66877985699920828 ) ) ;
#19963=CARTESIAN_POINT ( 'NONE',  ( -8.500000000000000000, 0.000000000000000000, -81.99999999999998579 ) ) ;
#19967=DIRECTION ( 'NONE',  ( 0.000000000000000000, 0.000000000000000000, 1.000000000000000000 ) ) ;
#19974=EDGE_CURVE ( 'NONE', #15733, #9763, #17184, .T. ) ;
#19975=CARTESIAN_POINT ( 'NONE',  ( 30.00000000000000000, -50.00000000000000000, 66.88656633939929463 ) ) ;
#19980=CARTESIAN_POINT ( 'NONE',  ( -13.12108515385492247, -17.04513403132573046, 78.38820092699481279 ) ) ;
#19984=EDGE_CURVE ( 'NONE', #8060, #8274, #2957, .T. ) ;
#19986=CARTESIAN_POINT ( 'NONE',  ( 30.06717155927020713, -106.8759708378635054, 77.91277504389037745 ) ) ;
#19987=CARTESIAN_POINT ( 'NONE',  ( 42.29298993630181513, -123.8503867192492578, -81.55043513968610114 ) ) ;
#19990=ORIENTED_EDGE ( 'NONE', *, *, #19805, .F. ) ;
#19996=AXIS2_PLACEMENT_3D ( 'NONE', #13181, #5018, #6702 ) ;
#19997=CARTESIAN_POINT ( 'NONE',  ( -24.99999999999999289, -170.8299878242309546, 15.48896927112552824 ) ) ;
#20013=AXIS2_PLACEMENT_3D ( 'NONE', #14424, #5251, #17912 ) ;
#20016=EDGE_LOOP ( 'NONE', ( #4242, #1985 ) ) ;
#20017=DIRECTION ( 'NONE',  ( 0.000000000000000000, -0.000000000000000000, -1.000000000000000000 ) ) ;
#20018=CARTESIAN_POINT ( 'NONE',  ( 38.45380490109781135, -18.24950758230019332, -72.03149080720356778 ) ) ;
#20020=AXIS2_PLACEMENT_3D ( 'NONE', #19858, #10003, #3051 ) ;
#20027=EDGE_CURVE ( 'NONE', #834, #15340, #4300, .T. ) ;
#20030=CARTESIAN_POINT ( 'NONE',  ( 30.00000000000000000, -99.99999999999998579, -52.00000000000000000 ) ) ;
#20038=CARTESIAN_POINT ( 'NONE',  ( -19.43057967899845551, -9.208910241125163765, 77.65734690581830080 ) ) ;
#20048=ORIENTED_EDGE ( 'NONE', *, *, #7956, .T. ) ;
#20051=CARTESIAN_POINT ( 'NONE',  ( -30.00000000000000000, -40.00000000000000000, -130.0000000000000000 ) ) ;
#20053=CARTESIAN_POINT ( 'NONE',  ( 30.00000000000000000, -50.00000000000000000, -66.88656633939928042 ) ) ;
#20056=CIRCLE ( 'NONE', #6199, 21.50000000000000000 ) ;
#20060=CARTESIAN_POINT ( 'NONE',  ( 18.13963350654227469, -26.35784117651622793, -130.0000000000000000 ) ) ;
#20062=CARTESIAN_POINT ( 'NONE',  ( 19.54001732319277096, -8.991134644608420601, -77.82005195698282307 ) ) ;
#20063=ADVANCED_FACE ( 'NONE', ( #17465 ), #20303, .T. ) ;
#20068=FACE_OUTER_BOUND ( 'NONE', #9988, .T. ) ;
#20069=AXIS2_PLACEMENT_3D ( 'NONE', #14833, #13235, #11341 ) ;
#20070=ORIENTED_EDGE ( 'NONE', *, *, #3343, .F. ) ;
#20072=EDGE_LOOP ( 'NONE', ( #17311, #6464, #20644, #16353 ) ) ;
#20075=VERTEX_POINT ( 'NONE', #4416 ) ;
#20077=DIRECTION ( 'NONE',  ( 0.000000000000000000, 0.000000000000000000, -1.000000000000000000 ) ) ;
#20078=CIRCLE ( 'NONE', #12318, 8.999999999999994671 ) ;
#20088=CARTESIAN_POINT ( 'NONE',  ( -14.15758254428918228, -16.19451531421082535, 78.90478163254508104 ) ) ;
#20091=VECTOR ( 'NONE', #13082, 1000.000000000000000 ) ;
#20094=EDGE_LOOP ( 'NONE', ( #14623, #17843, #1976, #1361 ) ) ;
#20100=CARTESIAN_POINT ( 'NONE',  ( 3.105127573534534502, -22.79270295337239105, -75.46210090792683900 ) ) ;
#20104=ORIENTED_EDGE ( 'NONE', *, *, #10266, .T. ) ;
#20106=CYLINDRICAL_SURFACE ( 'NONE', #17499, 5.000000000000004441 ) ;
#20111=EDGE_CURVE ( 'NONE', #13834, #10203, #16491, .T. ) ;
#20113=EDGE_CURVE ( 'NONE', #2104, #12463, #10685, .T. ) ;
#20121=VECTOR ( 'NONE', #6205, 1000.000000000000000 ) ;
#20122=ORIENTED_EDGE ( 'NONE', *, *, #12990, .F. ) ;
#20127=DIRECTION ( 'NONE',  ( -1.000000000000000000, 0.000000000000000000, 0.000000000000000000 ) ) ;
#20130=CARTESIAN_POINT ( 'NONE',  ( -39.99999999999999289, -30.00000000000000000, -130.0000000000000000 ) ) ;
#20136=CYLINDRICAL_SURFACE ( 'NONE', #10973, 5.000000000000004441 ) ;
#20138=CARTESIAN_POINT ( 'NONE',  ( 0.000000000000000000, 0.000000000000000000, -90.00000000000000000 ) ) ;
#20146=CARTESIAN_POINT ( 'NONE',  ( -21.39626923676110692, -2.341574137301850822, 83.84978971573227113 ) ) ;
#20149=DIRECTION ( 'NONE',  ( -0.000000000000000000, -3.469446951953614682E-16, -1.000000000000000000 ) ) ;
#20150=ORIENTED_EDGE ( 'NONE', *, *, #17562, .T. ) ;
#20156=ORIENTED_EDGE ( 'NONE', *, *, #820, .F. ) ;
#20160=DIRECTION ( 'NONE',  ( 0.000000000000000000, 0.000000000000000000, -1.000000000000000000 ) ) ;
#20166=CIRCLE ( 'NONE', #16786, 10.00000000000000178 ) ;
#20172=CARTESIAN_POINT ( 'NONE',  ( 1.457308041610593241, -21.46427008073574783, -70.59507481315787913 ) ) ;
#20173=ORIENTED_EDGE ( 'NONE', *, *, #3395, .T. ) ;
#20175=VECTOR ( 'NONE', #17423, 1000.000000000000000 ) ;
#20180=CIRCLE ( 'NONE', #1601, 20.00000000000000000 ) ;
#20181=ORIENTED_EDGE ( 'NONE', *, *, #12317, .F. ) ;
#20184=AXIS2_PLACEMENT_3D ( 'NONE', #15237, #7177, #3996 ) ;
#20188=AXIS2_PLACEMENT_3D ( 'NONE', #13838, #15107, #16797 ) ;
#20192=CYLINDRICAL_SURFACE ( 'NONE', #767, 75.00000000000000000 ) ;
#20195=ORIENTED_EDGE ( 'NONE', *, *, #4677, .F. ) ;
#20198=EDGE_CURVE ( 'NONE', #9451, #18686, #13790, .T. ) ;
#20201=AXIS2_PLACEMENT_3D ( 'NONE', #7380, #12699, #13856 ) ;
#20206=CARTESIAN_POINT ( 'NONE',  ( 30.00000000000000000, -99.99999999999998579, 49.90000000000000568 ) ) ;
#20209=CARTESIAN_POINT ( 'NONE',  ( 30.00000000000000000, -85.00000000000000000, -1.040949779275250179E-14 ) ) ;
#20216=CARTESIAN_POINT ( 'NONE',  ( 48.35276434571220250, -3.649167310370807105, -90.00000000000000000 ) ) ;
#20220=EDGE_CURVE ( 'NONE', #12782, #15733, #8220, .T. ) ;
#20232=FACE_OUTER_BOUND ( 'NONE', #16976, .T. ) ;
#20236=CARTESIAN_POINT ( 'NONE',  ( 50.00000000000000000, -42.57363661491096707, 121.3828884801879155 ) ) ;
#20241=VERTEX_POINT ( 'NONE', #11411 ) ;
#20246=CARTESIAN_POINT ( 'NONE',  ( 50.00000000000000000, -3.649167310370807105, -90.00000000000000000 ) ) ;
#20254=LINE ( 'NONE', #6154, #13063 ) ;
#20257=EDGE_LOOP ( 'NONE', ( #2146, #2706, #5445, #2426 ) ) ;
#20259=CARTESIAN_POINT ( 'NONE',  ( 13.80207632871711532, -16.50074880709951586, 72.95245019206022619 ) ) ;
#20264=CARTESIAN_POINT ( 'NONE',  ( 0.000000000000000000, 0.000000000000000000, 84.99999999999998579 ) ) ;
#20265=CARTESIAN_POINT ( 'NONE',  ( 50.00000000000000000, -159.9999999999999716, 53.99496054166690584 ) ) ;
#20277=CARTESIAN_POINT ( 'NONE',  ( -3.872723063507617525, -21.16211945945224571, -70.72147569179591642 ) ) ;
#20281=PLANE ( 'NONE',  #2938 ) ;
#20282=VERTEX_POINT ( 'NONE', #3445 ) ;
#20285=DIRECTION ( 'NONE',  ( 0.000000000000000000, 0.000000000000000000, -1.000000000000000000 ) ) ;
#20286=VERTEX_POINT ( 'NONE', #4735 ) ;
#20298=DIRECTION ( 'NONE',  ( -1.000000000000000000, 0.000000000000000000, 0.000000000000000000 ) ) ;
#20300=EDGE_CURVE ( 'NONE', #14747, #16465, #19156, .T. ) ;
#20303=PLANE ( 'NONE',  #15808 ) ;
#20307=CARTESIAN_POINT ( 'NONE',  ( 18.08416879489398355, -14.22778436779400124, -80.18931099398717777 ) ) ;
#20308=EDGE_LOOP ( 'NONE', ( #13956, #17459, #6448, #307, #12204, #20312 ) ) ;
#20312=ORIENTED_EDGE ( 'NONE', *, *, #7957, .F. ) ;
#20316=PLANE ( 'NONE',  #19024 ) ;
#20317=DIRECTION ( 'NONE',  ( 0.000000000000000000, 0.000000000000000000, -1.000000000000000000 ) ) ;
#20329=ADVANCED_FACE ( 'NONE', ( #883, #2683 ), #19656, .F. ) ;
#20335=CARTESIAN_POINT ( 'NONE',  ( 36.39485347990547837, -22.16933930360253768, -75.72923816920850015 ) ) ;
#20337=VERTEX_POINT ( 'NONE', #8929 ) ;
#20339=EDGE_CURVE ( 'NONE', #17908, #15704, #7694, .T. ) ;
#20352=VECTOR ( 'NONE', #2528, 1000.000000000000000 ) ;
#20362=CARTESIAN_POINT ( 'NONE',  ( 21.39608139526260899, -2.344611746178262734, 83.84634603192272095 ) ) ;
#20365=DIRECTION ( 'NONE',  ( 0.000000000000000000, 0.000000000000000000, 1.000000000000000000 ) ) ;
#20368=CARTESIAN_POINT ( 'NONE',  ( 42.30813292954685068, -123.8249046810892082, 81.51046245632689136 ) ) ;
#20380=ORIENTED_EDGE ( 'NONE', *, *, #8821, .F. ) ;
#20383=LINE ( 'NONE', #18488, #5942 ) ;
#20387=CARTESIAN_POINT ( 'NONE',  ( -19.00859264729083620, -10.06624177801187869, -77.01193977728050299 ) ) ;
#20394=AXIS2_PLACEMENT_3D ( 'NONE', #14525, #3176, #6352 ) ;
#20395=DIRECTION ( 'NONE',  ( -1.000000000000000000, 0.000000000000000000, 0.000000000000000000 ) ) ;
#20396=FACE_BOUND ( 'NONE', #11478, .T. ) ;
#20406=CARTESIAN_POINT ( 'NONE',  ( 30.00000000000000000, -50.00000000000000000, 71.93747284969079203 ) ) ;
#20409=EDGE_LOOP ( 'NONE', ( #17914, #17756, #17778, #7247 ) ) ;
#20413=CARTESIAN_POINT ( 'NONE',  ( -14.65527575808362037, -15.74483652605746009, 79.18672471502033261 ) ) ;
#20420=EDGE_LOOP ( 'NONE', ( #10446, #11640, #11615, #1924 ) ) ;
#20421=DIRECTION ( 'NONE',  ( 1.000000000000000000, 0.000000000000000000, 0.000000000000000000 ) ) ;
#20425=CARTESIAN_POINT ( 'NONE',  ( 22.32918011041974893, -5.620274625700770521, -87.66817617122062245 ) ) ;
#20427=CARTESIAN_POINT ( 'NONE',  ( -30.00000000000000000, 36.35083268962915781, 50.00000000000000000 ) ) ;
#20430=ORIENTED_EDGE ( 'NONE', *, *, #2739, .F. ) ;
#20432=ORIENTED_EDGE ( 'NONE', *, *, #17750, .T. ) ;
#20433=DIRECTION ( 'NONE',  ( 0.000000000000000000, 0.000000000000000000, -1.000000000000000000 ) ) ;
#20441=CIRCLE ( 'NONE', #19104, 3.199999999999994404 ) ;
#20453=ORIENTED_EDGE ( 'NONE', *, *, #12703, .T. ) ;
#20455=VERTEX_POINT ( 'NONE', #19769 ) ;
#20463=ADVANCED_FACE ( 'NONE', ( #18190, #2069 ), #8523, .F. ) ;
#20469=DIRECTION ( 'NONE',  ( 0.000000000000000000, 1.040834085586084454E-15, -1.000000000000000000 ) ) ;
#20470=ADVANCED_FACE ( 'NONE', ( #14348 ), #17309, .F. ) ;
#20473=EDGE_LOOP ( 'NONE', ( #11668, #15089, #13911, #12138 ) ) ;
#20475=DIRECTION ( 'NONE',  ( 0.000000000000000000, 0.000000000000000000, 1.000000000000000000 ) ) ;
#20478=DIRECTION ( 'NONE',  ( -0.000000000000000000, -0.000000000000000000, 1.000000000000000000 ) ) ;
#20483=ORIENTED_EDGE ( 'NONE', *, *, #6089, .T. ) ;
#20495=ADVANCED_FACE ( 'NONE', ( #9357 ), #1318, .F. ) ;
#20497=ORIENTED_EDGE ( 'NONE', *, *, #17866, .F. ) ;
#20498=DIRECTION ( 'NONE',  ( 1.000000000000000000, 0.000000000000000000, 0.000000000000000000 ) ) ;
#20504=DIRECTION ( 'NONE',  ( 0.000000000000000000, 0.000000000000000000, 1.000000000000000000 ) ) ;
#20512=CARTESIAN_POINT ( 'NONE',  ( 33.22510083995761221, -115.8989469114827955, 76.12820955576133031 ) ) ;
#20526=CARTESIAN_POINT ( 'NONE',  ( 43.62500077266425791, -125.0000000000000000, 90.00000000000002842 ) ) ;
#20527=CIRCLE ( 'NONE', #7671, 11.50000000000000000 ) ;
#20532=VERTEX_POINT ( 'NONE', #2784 ) ;
#20533=FACE_OUTER_BOUND ( 'NONE', #18065, .T. ) ;
#20537=VERTEX_POINT ( 'NONE', #9252 ) ;
#20538=DIRECTION ( 'NONE',  ( 1.000000000000000000, 0.000000000000000000, 0.000000000000000000 ) ) ;
#20549=DIRECTION ( 'NONE',  ( 0.000000000000000000, -1.040834085586084454E-15, 1.000000000000000000 ) ) ;
#20553=FACE_OUTER_BOUND ( 'NONE', #6913, .T. ) ;
#20558=DIRECTION ( 'NONE',  ( 0.000000000000000000, 0.000000000000000000, -1.000000000000000000 ) ) ;
#20563=CARTESIAN_POINT ( 'NONE',  ( 39.31722773736984067, -16.79517646696619693, -78.51518414706339399 ) ) ;
#20567=VERTEX_POINT ( 'NONE', #3096 ) ;
#20568=CARTESIAN_POINT ( 'NONE',  ( 30.97876637327306071, -111.1959070590765748, -74.06233646255252268 ) ) ;
#20577=DIRECTION ( 'NONE',  ( 1.000000000000000000, -0.000000000000000000, -0.000000000000000000 ) ) ;
#20580=ORIENTED_EDGE ( 'NONE', *, *, #20607, .F. ) ;
#20582=CARTESIAN_POINT ( 'NONE',  ( 18.66082225198899636, -10.69875493221384311, 76.55584491636111011 ) ) ;
#20594=CARTESIAN_POINT ( 'NONE',  ( 50.00000000000000000, -170.8299878242309546, -15.48896927112552824 ) ) ;
#20596=EDGE_LOOP ( 'NONE', ( #6686, #15928 ) ) ;
#20607=EDGE_CURVE ( 'NONE', #6801, #14238, #7707, .T. ) ;
#20612=VERTEX_POINT ( 'NONE', #9001 ) ;
#20614=DIRECTION ( 'NONE',  ( 0.000000000000000000, -1.000000000000000000, -0.000000000000000000 ) ) ;
#20621=CARTESIAN_POINT ( 'NONE',  ( 17.89279294550298260, -11.93604557640007613, 81.86420770708537020 ) ) ;
#20630=CARTESIAN_POINT ( 'NONE',  ( 24.99999999999999289, -30.00000000000000711, 44.99999999999998579 ) ) ;
#20638=CARTESIAN_POINT ( 'NONE',  ( 30.00000000000000000, -85.00000000000000000, -1.040949779275250179E-14 ) ) ;
#20644=ORIENTED_EDGE ( 'NONE', *, *, #18534, .T. ) ;
#20655=VERTEX_POINT ( 'NONE', #844 ) ;
#20660=EDGE_LOOP ( 'NONE', ( #2083, #3561, #13260, #4527, #18786 ) ) ;
#20661=CARTESIAN_POINT ( 'NONE',  ( 39.99999999999997158, -122.3205080756887497, -80.28096411455980785 ) ) ;
#20668=CARTESIAN_POINT ( 'NONE',  ( 10.00000000000000178, -160.0000000000000000, 70.00000000000000000 ) ) ;
#20675=CARTESIAN_POINT ( 'NONE',  ( 30.00000000000000000, 4.299168419249259188, -90.00000000000000000 ) ) ;
#20677=ORIENTED_EDGE ( 'NONE', *, *, #5772, .T. ) ;
#20680=CARTESIAN_POINT ( 'NONE',  ( -21.35784117651625280, 26.35784117651607872, -120.0000000000000142 ) ) ;
#20684=DIRECTION ( 'NONE',  ( 0.000000000000000000, 0.000000000000000000, 1.000000000000000000 ) ) ;
#20695=EDGE_LOOP ( 'NONE', ( #4927, #8554, #19490, #3630, #17965 ) ) ;
#20697=CARTESIAN_POINT ( 'NONE',  ( 50.00100000000000477, -85.00000000000000000, -9.000000000000005329 ) ) ;
#20698=CARTESIAN_POINT ( 'NONE',  ( -11.50000000000000000, 0.000000000000000000, -68.00000000000000000 ) ) ;
#20704=VERTEX_POINT ( 'NONE', #9109 ) ;
#20710=ORIENTED_EDGE ( 'NONE', *, *, #14277, .T. ) ;
#20721=CARTESIAN_POINT ( 'NONE',  ( 9.580208064738101825, -19.26033094913555388, 77.14905570196101792 ) ) ;
#20725=VERTEX_POINT ( 'NONE', #6031 ) ;
#20731=LINE ( 'NONE', #12587, #3104 ) ;
#20734=VECTOR ( 'NONE', #15449, 1000.000000000000000 ) ;
#20739=CARTESIAN_POINT ( 'NONE',  ( 40.00000000000000000, -122.3205080756887639, 86.97287527660684248 ) ) ;
#20746=ORIENTED_EDGE ( 'NONE', *, *, #6746, .F. ) ;
#20751=EDGE_CURVE ( 'NONE', #2701, #5755, #8043, .T. ) ;
#20752=VERTEX_POINT ( 'NONE', #14412 ) ;
#20756=AXIS2_PLACEMENT_3D ( 'NONE', #11529, #3373, #14621 ) ;
#20761=CARTESIAN_POINT ( 'NONE',  ( -24.99999999999999289, -85.00000000000000000, 8.999999999999984013 ) ) ;
#20764=EDGE_CURVE ( 'NONE', #11513, #8121, #18538, .T. ) ;
#20766=DIRECTION ( 'NONE',  ( -1.000000000000000000, 0.000000000000000000, 0.000000000000000000 ) ) ;
#20767=VECTOR ( 'NONE', #1833, 1000.000000000000000 ) ;
#20778=AXIS2_PLACEMENT_3D ( 'NONE', #17689, #3159, #6842 ) ;
#20784=ORIENTED_EDGE ( 'NONE', *, *, #6504, .F. ) ;
#20791=ORIENTED_EDGE ( 'NONE', *, *, #7181, .T. ) ;
#20795=CIRCLE ( 'NONE', #8262, 35.00000000000000000 ) ;
#20796=EDGE_LOOP ( 'NONE', ( #13348, #14388, #9167, #14855 ) ) ;
#20805=VERTEX_POINT ( 'NONE', #4747 ) ;
#20809=ADVANCED_FACE ( 'NONE', ( #1686 ), #17377, .F. ) ;
#20820=VERTEX_POINT ( 'NONE', #6235 ) ;
#20821=DIRECTION ( 'NONE',  ( 0.000000000000000000, 0.000000000000000000, 1.000000000000000000 ) ) ;
#20841=CARTESIAN_POINT ( 'NONE',  ( -22.32752340640299238, -5.629990940594709947, -87.65661170390809787 ) ) ;
#20843=CARTESIAN_POINT ( 'NONE',  ( -21.50000000000000000, 0.000000000000000000, -68.00000000000000000 ) ) ;
#20845=ORIENTED_EDGE ( 'NONE', *, *, #4835, .T. ) ;
#20861=DIRECTION ( 'NONE',  ( -1.000000000000000000, -0.000000000000000000, -0.000000000000000000 ) ) ;
#20862=CARTESIAN_POINT ( 'NONE',  ( 37.34030720104099998, -20.29716165210874479, 71.08834080262353439 ) ) ;
#20865=CYLINDRICAL_SURFACE ( 'NONE', #20394, 2.099999999999997868 ) ;
#20867=ORIENTED_EDGE ( 'NONE', *, *, #274, .F. ) ;
#20874=CARTESIAN_POINT ( 'NONE',  ( 30.25369199320016023, -108.6370530507956289, -73.18626058406910317 ) ) ;
#20875=CIRCLE ( 'NONE', #15112, 80.00000000000000000 ) ;
#20885=CYLINDRICAL_SURFACE ( 'NONE', #17658, 11.49999999999999645 ) ;
#20890=ORIENTED_EDGE ( 'NONE', *, *, #19573, .F. ) ;
#20893=ORIENTED_EDGE ( 'NONE', *, *, #7035, .T. ) ;
#20895=DIRECTION ( 'NONE',  ( 1.000000000000000000, -0.000000000000000000, -0.000000000000000000 ) ) ;
#20900=DIRECTION ( 'NONE',  ( 0.000000000000000000, 0.000000000000000000, 1.000000000000000000 ) ) ;
#20919=CARTESIAN_POINT ( 'NONE',  ( -24.99999999999999289, -85.00000000000000000, -1.040949779275250179E-14 ) ) ;
#20926=CARTESIAN_POINT ( 'NONE',  ( 30.00000000000000355, -139.6410161513775563, -90.00000000000001421 ) ) ;
#20927=ADVANCED_FACE ( 'NONE', ( #5365, #9824, #10042, #391, #11430, #14714 ), #6741, .T. ) ;
ENDSEC;
END-ISO-10303-21;
